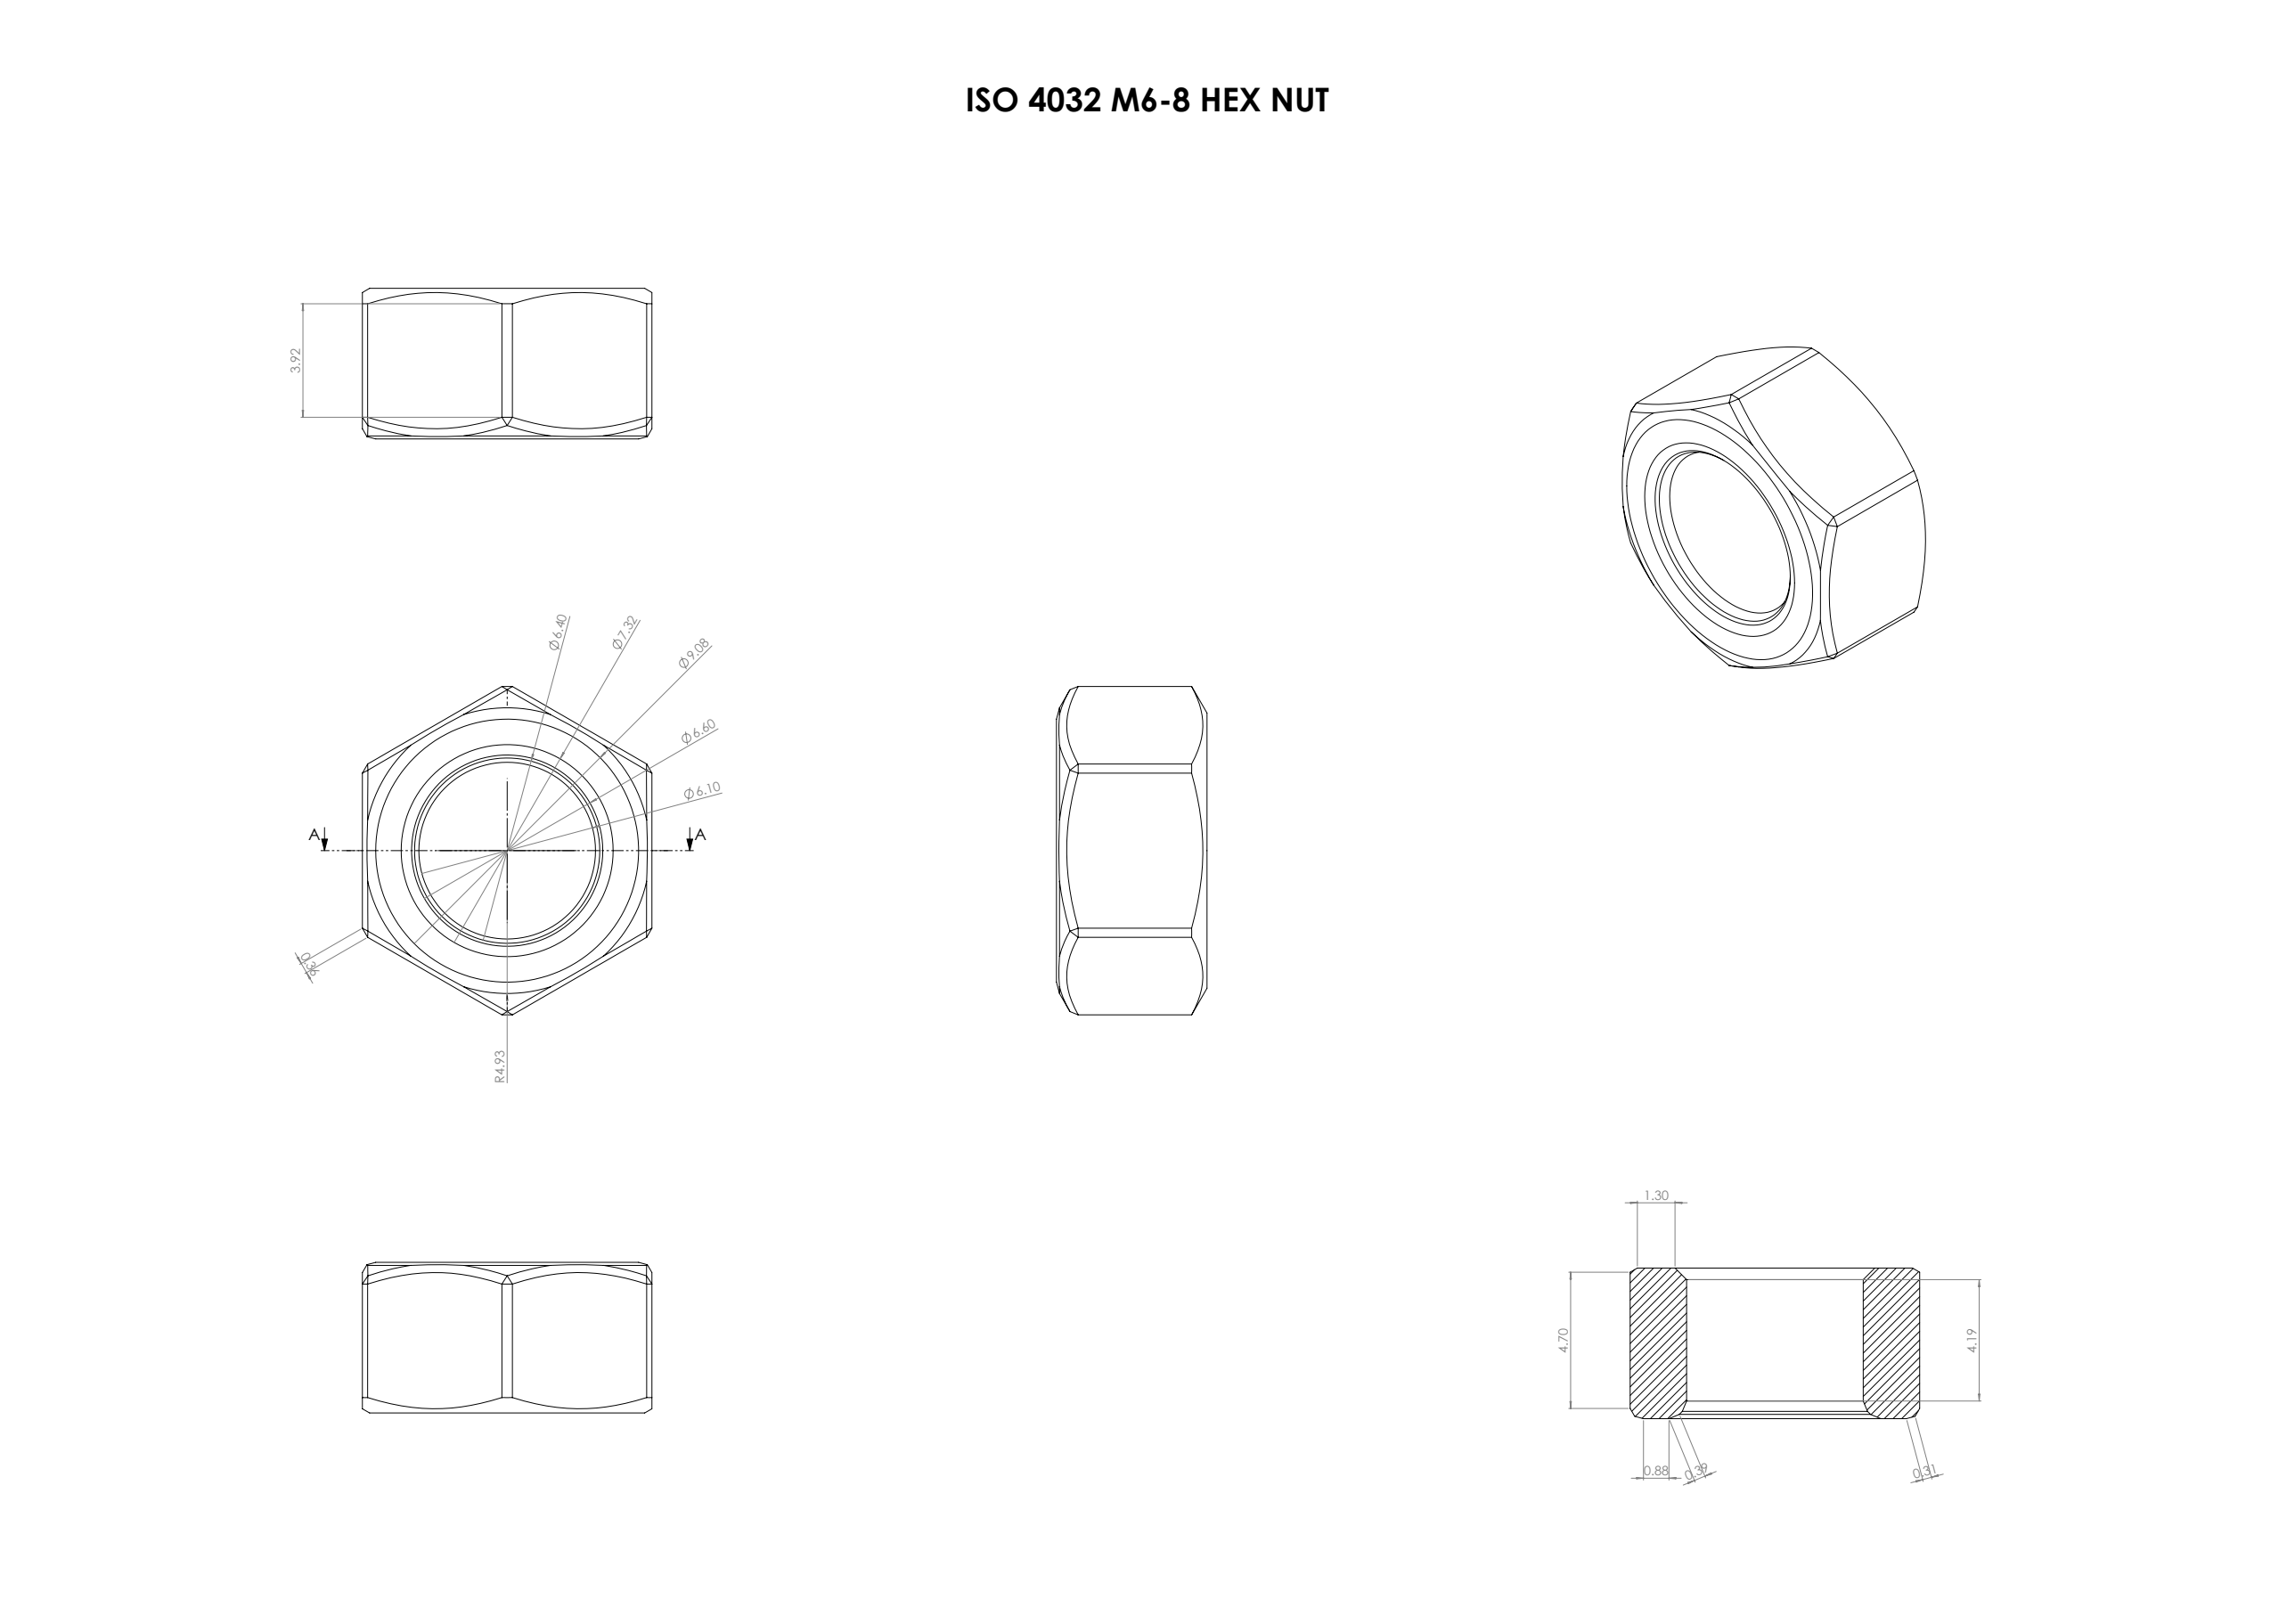
ISO-10303-21;
HEADER;
/* Generated by software containing ST-Developer
 * from STEP Tools, Inc. (www.steptools.com) 
 */

FILE_DESCRIPTION(
/* description */ (''),
/* implementation_level */ '2;1');

FILE_NAME(
/* name */ 
'11_ISO_4032_M6-8_Hex_Nut.step',
/* time_stamp */ '2026-10-22T00:21:42-07:00',
/* author */ (''),
/* organization */ (''),
/* preprocessor_version */ 'ST-DEVELOPER v20.2',
/* originating_system */ 'Autodesk Translation Framework v15.15.0.0',
/* authorisation */ '');

FILE_SCHEMA (('AUTOMOTIVE_DESIGN { 1 0 10303 214 3 1 1 }'));
ENDSEC;

DATA;
#10=MECHANICAL_DESIGN_GEOMETRIC_PRESENTATION_REPRESENTATION('',(#215),#31638);
#159=(
BOUNDED_CURVE()
B_SPLINE_CURVE(2,(#31154,#31155,#31156),.UNSPECIFIED.,.F.,.F.)
B_SPLINE_CURVE_WITH_KNOTS((3,3),(0.0913980941282311,0.128154684519473),
 .UNSPECIFIED.)
CURVE()
GEOMETRIC_REPRESENTATION_ITEM()
RATIONAL_B_SPLINE_CURVE((1.009002117709,1.00952129238835,1.009002117709))
REPRESENTATION_ITEM('')
);
#160=(
BOUNDED_CURVE()
B_SPLINE_CURVE(2,(#31282,#31283,#31284),.UNSPECIFIED.,.F.,.F.)
B_SPLINE_CURVE_WITH_KNOTS((3,3),(0.0913980941282308,0.128154684519473),
 .UNSPECIFIED.)
CURVE()
GEOMETRIC_REPRESENTATION_ITEM()
RATIONAL_B_SPLINE_CURVE((1.009002117709,1.00952129238836,1.009002117709))
REPRESENTATION_ITEM('')
);
#161=(
BOUNDED_CURVE()
B_SPLINE_CURVE(2,(#31290,#31291,#31292),.UNSPECIFIED.,.F.,.F.)
B_SPLINE_CURVE_WITH_KNOTS((3,3),(0.0913980941282322,0.128154684519474),
 .UNSPECIFIED.)
CURVE()
GEOMETRIC_REPRESENTATION_ITEM()
RATIONAL_B_SPLINE_CURVE((1.009002117709,1.00952129238836,1.009002117709))
REPRESENTATION_ITEM('')
);
#162=(
BOUNDED_CURVE()
B_SPLINE_CURVE(2,(#31423,#31424,#31425),.UNSPECIFIED.,.F.,.F.)
B_SPLINE_CURVE_WITH_KNOTS((3,3),(0.0913980941282321,0.128154684519474),
 .UNSPECIFIED.)
CURVE()
GEOMETRIC_REPRESENTATION_ITEM()
RATIONAL_B_SPLINE_CURVE((1.009002117709,1.00952129238835,1.009002117709))
REPRESENTATION_ITEM('')
);
#163=(
BOUNDED_CURVE()
B_SPLINE_CURVE(2,(#31431,#31432,#31433),.UNSPECIFIED.,.F.,.F.)
B_SPLINE_CURVE_WITH_KNOTS((3,3),(0.0913980941282314,0.128154684519474),
 .UNSPECIFIED.)
CURVE()
GEOMETRIC_REPRESENTATION_ITEM()
RATIONAL_B_SPLINE_CURVE((1.00900211770901,1.00952129238836,1.00900211770901))
REPRESENTATION_ITEM('')
);
#164=(
BOUNDED_CURVE()
B_SPLINE_CURVE(2,(#31499,#31500,#31501),.UNSPECIFIED.,.F.,.F.)
B_SPLINE_CURVE_WITH_KNOTS((3,3),(0.0913980941282296,0.128154684519472),
 .UNSPECIFIED.)
CURVE()
GEOMETRIC_REPRESENTATION_ITEM()
RATIONAL_B_SPLINE_CURVE((1.00900211770901,1.00952129238837,1.00900211770901))
REPRESENTATION_ITEM('')
);
#165=(
BOUNDED_CURVE()
B_SPLINE_CURVE(2,(#31505,#31506,#31507),.UNSPECIFIED.,.F.,.F.)
B_SPLINE_CURVE_WITH_KNOTS((3,3),(0.0979198359865813,0.674024179098759),
 .UNSPECIFIED.)
CURVE()
GEOMETRIC_REPRESENTATION_ITEM()
RATIONAL_B_SPLINE_CURVE((1.0564201716687,1.19828036671056,1.0564201716687))
REPRESENTATION_ITEM('')
);
#166=(
BOUNDED_CURVE()
B_SPLINE_CURVE(2,(#31509,#31510,#31511),.UNSPECIFIED.,.F.,.F.)
B_SPLINE_CURVE_WITH_KNOTS((3,3),(0.0979198359865817,0.674024179098759),
 .UNSPECIFIED.)
CURVE()
GEOMETRIC_REPRESENTATION_ITEM()
RATIONAL_B_SPLINE_CURVE((1.0564201716687,1.19828036671056,1.0564201716687))
REPRESENTATION_ITEM('')
);
#167=(
BOUNDED_CURVE()
B_SPLINE_CURVE(2,(#31513,#31514,#31515),.UNSPECIFIED.,.F.,.F.)
B_SPLINE_CURVE_WITH_KNOTS((3,3),(0.0979198359865813,0.674024179098759),
 .UNSPECIFIED.)
CURVE()
GEOMETRIC_REPRESENTATION_ITEM()
RATIONAL_B_SPLINE_CURVE((1.0564201716687,1.19828036671056,1.0564201716687))
REPRESENTATION_ITEM('')
);
#168=(
BOUNDED_CURVE()
B_SPLINE_CURVE(2,(#31521,#31522,#31523),.UNSPECIFIED.,.F.,.F.)
B_SPLINE_CURVE_WITH_KNOTS((3,3),(0.0979198359865812,0.385972007542669),
 .UNSPECIFIED.)
CURVE()
GEOMETRIC_REPRESENTATION_ITEM()
RATIONAL_B_SPLINE_CURVE((1.0564201716687,1.12735026918963,1.12735026918963))
REPRESENTATION_ITEM('')
);
#169=(
BOUNDED_CURVE()
B_SPLINE_CURVE(2,(#31524,#31525,#31526),.UNSPECIFIED.,.F.,.F.)
B_SPLINE_CURVE_WITH_KNOTS((3,3),(0.0979198359865812,0.674024179098759),
 .UNSPECIFIED.)
CURVE()
GEOMETRIC_REPRESENTATION_ITEM()
RATIONAL_B_SPLINE_CURVE((1.0564201716687,1.19828036671056,1.0564201716687))
REPRESENTATION_ITEM('')
);
#170=(
BOUNDED_CURVE()
B_SPLINE_CURVE(2,(#31527,#31528,#31529),.UNSPECIFIED.,.F.,.F.)
B_SPLINE_CURVE_WITH_KNOTS((3,3),(0.0979198359865813,0.674024179098759),
 .UNSPECIFIED.)
CURVE()
GEOMETRIC_REPRESENTATION_ITEM()
RATIONAL_B_SPLINE_CURVE((1.0564201716687,1.19828036671056,1.0564201716687))
REPRESENTATION_ITEM('')
);
#171=(
BOUNDED_CURVE()
B_SPLINE_CURVE(2,(#31530,#31531,#31532),.UNSPECIFIED.,.F.,.F.)
B_SPLINE_CURVE_WITH_KNOTS((3,3),(0.385972007542669,0.674024179098759),
 .UNSPECIFIED.)
CURVE()
GEOMETRIC_REPRESENTATION_ITEM()
RATIONAL_B_SPLINE_CURVE((1.12735026918963,1.12735026918963,1.0564201716687))
REPRESENTATION_ITEM('')
);
#193=SHAPE_REPRESENTATION_RELATIONSHIP('SRR','None',#31715,#204);
#204=ADVANCED_BREP_SHAPE_REPRESENTATION('',(#226),#31637);
#215=STYLED_ITEM('',(#31837),#226);
#226=MANIFOLD_SOLID_BREP('Hex nut',#12490);
#361=CYLINDRICAL_SURFACE('',#13575,0.305);
#445=CONICAL_SURFACE('',#13551,0.551175134594813,1.0471975511966);
#446=CONICAL_SURFACE('',#13553,0.551175134594813,1.0471975511966);
#447=CONICAL_SURFACE('',#13555,0.551175134594813,1.0471975511966);
#448=CONICAL_SURFACE('',#13557,0.551175134594813,1.0471975511966);
#449=CONICAL_SURFACE('',#13559,0.551175134594813,1.0471975511966);
#450=CONICAL_SURFACE('',#13561,0.551175134594813,1.0471975511966);
#451=CONICAL_SURFACE('',#13563,0.551175134594813,1.0471975511966);
#452=CONICAL_SURFACE('',#13565,0.473593266739736,1.30899693899575);
#453=CONICAL_SURFACE('',#13569,0.348075378797541,1.17809724509617);
#454=CONICAL_SURFACE('',#13571,0.325,0.785398163397448);
#455=CONICAL_SURFACE('',#13573,0.312424621202459,0.392699081698723);
#456=CONICAL_SURFACE('',#13577,0.325,0.785398163397448);
#1149=B_SPLINE_CURVE_WITH_KNOTS('',3,(#30994,#30995,#30996,#30997,#30998,
#30999),.UNSPECIFIED.,.F.,.F.,(4,2,4),(-0.0356445426705879,-0.017820065955887,
0.),.UNSPECIFIED.);
#1150=B_SPLINE_CURVE_WITH_KNOTS('',3,(#31000,#31001,#31002,#31003,#31004,
#31005),.UNSPECIFIED.,.F.,.F.,(4,2,4),(-0.0356445406593133,-0.0178242377363697,
0.),.UNSPECIFIED.);
#1151=B_SPLINE_CURVE_WITH_KNOTS('',3,(#31009,#31010,#31011,#31012,#31013,
#31014),.UNSPECIFIED.,.F.,.F.,(4,2,4),(-0.0356445426646998,-0.0178200659542505,
0.),.UNSPECIFIED.);
#1152=B_SPLINE_CURVE_WITH_KNOTS('',3,(#31016,#31017,#31018,#31019,#31020,
#31021),.UNSPECIFIED.,.F.,.F.,(4,2,4),(-0.0356445406608173,-0.0178242377372387,
0.),.UNSPECIFIED.);
#1153=B_SPLINE_CURVE_WITH_KNOTS('',3,(#31028,#31029,#31030,#31031,#31032,
#31033),.UNSPECIFIED.,.F.,.F.,(4,2,4),(-0.035644542668606,-0.0178200659552084,
0.),.UNSPECIFIED.);
#1154=B_SPLINE_CURVE_WITH_KNOTS('',3,(#31034,#31035,#31036,#31037,#31038,
#31039),.UNSPECIFIED.,.F.,.F.,(4,2,4),(-0.0356445406611976,-0.0178242377369016,
0.),.UNSPECIFIED.);
#1155=B_SPLINE_CURVE_WITH_KNOTS('',3,(#31043,#31044,#31045,#31046,#31047,
#31048),.UNSPECIFIED.,.F.,.F.,(4,2,4),(-0.0356445426695261,-0.0178200659558121,
0.),.UNSPECIFIED.);
#1156=B_SPLINE_CURVE_WITH_KNOTS('',3,(#31050,#31051,#31052,#31053,#31054,
#31055),.UNSPECIFIED.,.F.,.F.,(4,2,4),(-0.0356445406606661,-0.0178242377367645,
0.),.UNSPECIFIED.);
#1157=B_SPLINE_CURVE_WITH_KNOTS('',3,(#31062,#31063,#31064,#31065,#31066,
#31067),.UNSPECIFIED.,.F.,.F.,(4,2,4),(-0.0356445426677898,-0.0178200659551202,
0.),.UNSPECIFIED.);
#1158=B_SPLINE_CURVE_WITH_KNOTS('',3,(#31068,#31069,#31070,#31071,#31072,
#31073),.UNSPECIFIED.,.F.,.F.,(4,2,4),(-0.0356445406615696,-0.0178242377363734,
0.),.UNSPECIFIED.);
#1159=B_SPLINE_CURVE_WITH_KNOTS('',3,(#31077,#31078,#31079,#31080,#31081,
#31082),.UNSPECIFIED.,.F.,.F.,(4,2,4),(-0.0356445426680788,-0.017820065955108,
0.),.UNSPECIFIED.);
#1160=B_SPLINE_CURVE_WITH_KNOTS('',3,(#31084,#31085,#31086,#31087,#31088,
#31089),.UNSPECIFIED.,.F.,.F.,(4,2,4),(-0.0356445406623922,-0.0178242377374904,
0.),.UNSPECIFIED.);
#1161=B_SPLINE_CURVE_WITH_KNOTS('',3,(#31113,#31114,#31115,#31116,#31117,
#31118,#31119,#31120,#31121,#31122,#31123,#31124,#31125,#31126,#31127,#31128,
#31129,#31130,#31131,#31132,#31133,#31134,#31135,#31136,#31137),
 .UNSPECIFIED.,.F.,.F.,(4,3,3,3,3,3,3,3,4),(1.38777878078145E-17,0.0499520104369165,
0.0579096339663456,0.0689507685252385,0.0901012807338169,0.116325803406286,
0.146260951142593,0.196900647008064,0.212043967873001),.UNSPECIFIED.);
#1162=B_SPLINE_CURVE_WITH_KNOTS('',3,(#31138,#31139,#31140,#31141),
 .UNSPECIFIED.,.F.,.F.,(4,4),(0.50492078692473,0.681229914591334),
 .UNSPECIFIED.);
#1163=B_SPLINE_CURVE_WITH_KNOTS('',3,(#31142,#31143,#31144,#31145,#31146),
 .UNSPECIFIED.,.F.,.F.,(4,1,4),(-0.679321786705464,-0.343792306535718,-0.0926222283799249),
 .UNSPECIFIED.);
#1164=B_SPLINE_CURVE_WITH_KNOTS('',3,(#31147,#31148,#31149,#31150),
 .UNSPECIFIED.,.F.,.F.,(4,4),(0.0907141004940068,0.26702322816061),
 .UNSPECIFIED.);
#1165=B_SPLINE_CURVE_WITH_KNOTS('',3,(#31181,#31182,#31183,#31184,#31185,
#31186,#31187,#31188,#31189,#31190,#31191,#31192,#31193,#31194,#31195,#31196,
#31197,#31198,#31199,#31200,#31201,#31202,#31203,#31204,#31205),
 .UNSPECIFIED.,.F.,.F.,(4,3,3,3,3,3,3,3,4),(0.,0.0499552658273372,0.0579096339663306,
0.0689507685252128,0.0901012807337863,0.116325803406243,0.146260951142533,
0.196900647007959,0.212043967872853),.UNSPECIFIED.);
#1166=B_SPLINE_CURVE_WITH_KNOTS('',3,(#31206,#31207,#31208,#31209),
 .UNSPECIFIED.,.F.,.F.,(4,4),(0.504920786924729,0.681229914591334),
 .UNSPECIFIED.);
#1167=B_SPLINE_CURVE_WITH_KNOTS('',3,(#31210,#31211,#31212,#31213,#31214),
 .UNSPECIFIED.,.F.,.F.,(4,1,4),(-0.679321786705464,-0.343792306535718,-0.092622228379925),
 .UNSPECIFIED.);
#1168=B_SPLINE_CURVE_WITH_KNOTS('',3,(#31215,#31216,#31217,#31218),
 .UNSPECIFIED.,.F.,.F.,(4,4),(0.0907141004940068,0.26702322816061),
 .UNSPECIFIED.);
#1169=B_SPLINE_CURVE_WITH_KNOTS('',3,(#31241,#31242,#31243,#31244,#31245,
#31246,#31247,#31248,#31249,#31250,#31251,#31252,#31253,#31254,#31255,#31256,
#31257,#31258,#31259,#31260,#31261,#31262,#31263,#31264,#31265),
 .UNSPECIFIED.,.F.,.F.,(4,3,3,3,3,3,3,3,4),(0.,0.0499520104360042,0.0579096339663052,
0.0689507685251914,0.0901012807337567,0.116325803406213,0.14626095114252,
0.196900647008034,0.212043967872961),.UNSPECIFIED.);
#1170=B_SPLINE_CURVE_WITH_KNOTS('',3,(#31266,#31267,#31268,#31269),
 .UNSPECIFIED.,.F.,.F.,(4,4),(0.50492078692473,0.681229914591334),
 .UNSPECIFIED.);
#1171=B_SPLINE_CURVE_WITH_KNOTS('',3,(#31270,#31271,#31272,#31273,#31274),
 .UNSPECIFIED.,.F.,.F.,(4,1,4),(-0.679321786705465,-0.343792306535719,-0.092622228379925),
 .UNSPECIFIED.);
#1172=B_SPLINE_CURVE_WITH_KNOTS('',3,(#31275,#31276,#31277,#31278),
 .UNSPECIFIED.,.F.,.F.,(4,4),(0.0907141004940071,0.26702322816061),
 .UNSPECIFIED.);
#1173=B_SPLINE_CURVE_WITH_KNOTS('',3,(#31317,#31318,#31319,#31320,#31321,
#31322,#31323,#31324,#31325,#31326,#31327,#31328,#31329,#31330,#31331,#31332,
#31333,#31334,#31335,#31336,#31337,#31338,#31339,#31340,#31341),
 .UNSPECIFIED.,.F.,.F.,(4,3,3,3,3,3,3,3,4),(0.,0.0501067129681924,0.0579096339662997,
0.0901012807337445,0.116325803406229,0.14310556044029,0.146260951142586,
0.196900647008164,0.212043967873065),.UNSPECIFIED.);
#1174=B_SPLINE_CURVE_WITH_KNOTS('',3,(#31342,#31343,#31344,#31345),
 .UNSPECIFIED.,.F.,.F.,(4,4),(0.50492078692473,0.681229914591334),
 .UNSPECIFIED.);
#1175=B_SPLINE_CURVE_WITH_KNOTS('',3,(#31346,#31347,#31348,#31349,#31350),
 .UNSPECIFIED.,.F.,.F.,(4,1,4),(-0.679321786705464,-0.428151708549622,-0.0926222283799251),
 .UNSPECIFIED.);
#1176=B_SPLINE_CURVE_WITH_KNOTS('',3,(#31351,#31352,#31353,#31354),
 .UNSPECIFIED.,.F.,.F.,(4,4),(0.0907141004940069,0.267023228160609),
 .UNSPECIFIED.);
#1177=B_SPLINE_CURVE_WITH_KNOTS('',3,(#31377,#31378,#31379,#31380,#31381,
#31382,#31383,#31384,#31385,#31386,#31387,#31388,#31389),.UNSPECIFIED.,
 .F.,.F.,(4,3,3,3,4),(0.,0.050107747114841,0.0579096339663157,0.0901012807337753,
0.106028581745725),.UNSPECIFIED.);
#1178=B_SPLINE_CURVE_WITH_KNOTS('',3,(#31391,#31392,#31393,#31394,#31395,
#31396,#31397,#31398,#31399,#31400,#31401,#31402,#31403,#31404,#31405,#31406),
 .UNSPECIFIED.,.F.,.F.,(4,3,3,3,3,4),(0.106028581745725,0.11632580340628,
0.143105560440363,0.146260951142647,0.196900647008195,0.212043967873119),
 .UNSPECIFIED.);
#1179=B_SPLINE_CURVE_WITH_KNOTS('',3,(#31407,#31408,#31409,#31410),
 .UNSPECIFIED.,.F.,.F.,(4,4),(0.50492078692473,0.681229914591334),
 .UNSPECIFIED.);
#1180=B_SPLINE_CURVE_WITH_KNOTS('',3,(#31411,#31412,#31413,#31414,#31415),
 .UNSPECIFIED.,.F.,.F.,(4,1,4),(-0.679321786705464,-0.428151708549622,-0.0926222283799252),
 .UNSPECIFIED.);
#1181=B_SPLINE_CURVE_WITH_KNOTS('',3,(#31416,#31417,#31418,#31419),
 .UNSPECIFIED.,.F.,.F.,(4,4),(0.090714100494007,0.26702322816061),
 .UNSPECIFIED.);
#1182=B_SPLINE_CURVE_WITH_KNOTS('',3,(#31458,#31459,#31460,#31461,#31462,
#31463,#31464,#31465,#31466,#31467,#31468,#31469,#31470,#31471,#31472,#31473,
#31474,#31475,#31476,#31477,#31478,#31479,#31480,#31481,#31482),
 .UNSPECIFIED.,.F.,.F.,(4,3,3,3,3,3,3,3,4),(0.,0.0499520104361464,0.0579096339662874,
0.0689507685251644,0.0901012807337523,0.116325803406236,0.146260951142573,
0.196900647008118,0.21204396787299),.UNSPECIFIED.);
#1183=B_SPLINE_CURVE_WITH_KNOTS('',3,(#31483,#31484,#31485,#31486),
 .UNSPECIFIED.,.F.,.F.,(4,4),(0.504920786924729,0.681229914591334),
 .UNSPECIFIED.);
#1184=B_SPLINE_CURVE_WITH_KNOTS('',3,(#31487,#31488,#31489,#31490,#31491),
 .UNSPECIFIED.,.F.,.F.,(4,1,4),(-0.679321786705464,-0.343792306535719,-0.0926222283799251),
 .UNSPECIFIED.);
#1185=B_SPLINE_CURVE_WITH_KNOTS('',3,(#31492,#31493,#31494,#31495),
 .UNSPECIFIED.,.F.,.F.,(4,4),(0.0907141004940075,0.26702322816061),
 .UNSPECIFIED.);
#1334=B_SPLINE_SURFACE_WITH_KNOTS('',3,3,((#31091,#31092,#31093,#31094,
#31095),(#31096,#31097,#31098,#31099,#31100),(#31101,#31102,#31103,#31104,
#31105),(#31106,#31107,#31108,#31109,#31110)),.UNSPECIFIED.,.F.,.F.,.F.,
(4,4),(4,1,4),(0.,1.),(0.0907141004940068,0.343792306535718,0.681229914591334),
 .UNSPECIFIED.);
#1335=B_SPLINE_SURFACE_WITH_KNOTS('',3,3,((#31159,#31160,#31161,#31162,
#31163),(#31164,#31165,#31166,#31167,#31168),(#31169,#31170,#31171,#31172,
#31173),(#31174,#31175,#31176,#31177,#31178)),.UNSPECIFIED.,.F.,.F.,.F.,
(4,4),(4,1,4),(0.,1.),(0.0907141004940068,0.343792306535718,0.681229914591334),
 .UNSPECIFIED.);
#1336=B_SPLINE_SURFACE_WITH_KNOTS('',3,3,((#31219,#31220,#31221,#31222,
#31223),(#31224,#31225,#31226,#31227,#31228),(#31229,#31230,#31231,#31232,
#31233),(#31234,#31235,#31236,#31237,#31238)),.UNSPECIFIED.,.F.,.F.,.F.,
(4,4),(4,1,4),(0.,1.),(0.0907141004940071,0.343792306535719,0.681229914591334),
 .UNSPECIFIED.);
#1337=B_SPLINE_SURFACE_WITH_KNOTS('',3,3,((#31295,#31296,#31297,#31298,
#31299),(#31300,#31301,#31302,#31303,#31304),(#31305,#31306,#31307,#31308,
#31309),(#31310,#31311,#31312,#31313,#31314)),.UNSPECIFIED.,.F.,.F.,.F.,
(4,4),(4,1,4),(0.,1.),(0.0907141004940069,0.428151708549622,0.681229914591334),
 .UNSPECIFIED.);
#1338=B_SPLINE_SURFACE_WITH_KNOTS('',3,3,((#31355,#31356,#31357,#31358,
#31359),(#31360,#31361,#31362,#31363,#31364),(#31365,#31366,#31367,#31368,
#31369),(#31370,#31371,#31372,#31373,#31374)),.UNSPECIFIED.,.F.,.F.,.F.,
(4,4),(4,1,4),(0.,1.),(0.090714100494007,0.428151708549622,0.681229914591334),
 .UNSPECIFIED.);
#1339=B_SPLINE_SURFACE_WITH_KNOTS('',3,3,((#31436,#31437,#31438,#31439,
#31440),(#31441,#31442,#31443,#31444,#31445),(#31446,#31447,#31448,#31449,
#31450),(#31451,#31452,#31453,#31454,#31455)),.UNSPECIFIED.,.F.,.F.,.F.,
(4,4),(4,1,4),(0.,1.),(0.0907141004940075,0.343792306535719,0.681229914591334),
 .UNSPECIFIED.);
#1403=FACE_BOUND('',#3261,.T.);
#1404=FACE_BOUND('',#3268,.T.);
#1805=CIRCLE('',#13552,0.475);
#1806=CIRCLE('',#13554,0.493186533479473);
#1807=CIRCLE('',#13556,0.493186533479473);
#1808=CIRCLE('',#13558,0.493186533479473);
#1809=CIRCLE('',#13560,0.493186533479473);
#1810=CIRCLE('',#13562,0.493186533479473);
#1811=CIRCLE('',#13564,0.493186533479473);
#1812=CIRCLE('',#13566,0.454);
#1813=CIRCLE('',#13568,0.366);
#1814=CIRCLE('',#13570,0.330150757595083);
#1815=CIRCLE('',#13572,0.319849242404917);
#1816=CIRCLE('',#13574,0.305);
#1817=CIRCLE('',#13576,0.305);
#1818=CIRCLE('',#13578,0.345);
#2474=FACE_OUTER_BOUND('',#3231,.T.);
#2475=FACE_OUTER_BOUND('',#3232,.T.);
#2476=FACE_OUTER_BOUND('',#3233,.T.);
#2477=FACE_OUTER_BOUND('',#3234,.T.);
#2478=FACE_OUTER_BOUND('',#3235,.T.);
#2479=FACE_OUTER_BOUND('',#3236,.T.);
#2480=FACE_OUTER_BOUND('',#3237,.T.);
#2481=FACE_OUTER_BOUND('',#3238,.T.);
#2482=FACE_OUTER_BOUND('',#3239,.T.);
#2483=FACE_OUTER_BOUND('',#3240,.T.);
#2484=FACE_OUTER_BOUND('',#3241,.T.);
#2485=FACE_OUTER_BOUND('',#3242,.T.);
#2486=FACE_OUTER_BOUND('',#3243,.T.);
#2487=FACE_OUTER_BOUND('',#3244,.T.);
#2488=FACE_OUTER_BOUND('',#3245,.T.);
#2489=FACE_OUTER_BOUND('',#3246,.T.);
#2490=FACE_OUTER_BOUND('',#3247,.T.);
#2491=FACE_OUTER_BOUND('',#3248,.T.);
#2492=FACE_OUTER_BOUND('',#3249,.T.);
#2493=FACE_OUTER_BOUND('',#3250,.T.);
#2494=FACE_OUTER_BOUND('',#3251,.T.);
#2495=FACE_OUTER_BOUND('',#3252,.T.);
#2496=FACE_OUTER_BOUND('',#3253,.T.);
#2497=FACE_OUTER_BOUND('',#3254,.T.);
#2498=FACE_OUTER_BOUND('',#3255,.T.);
#2499=FACE_OUTER_BOUND('',#3256,.T.);
#2500=FACE_OUTER_BOUND('',#3257,.T.);
#2501=FACE_OUTER_BOUND('',#3258,.T.);
#2502=FACE_OUTER_BOUND('',#3259,.T.);
#2503=FACE_OUTER_BOUND('',#3260,.T.);
#2504=FACE_OUTER_BOUND('',#3262,.T.);
#2505=FACE_OUTER_BOUND('',#3263,.T.);
#2506=FACE_OUTER_BOUND('',#3264,.T.);
#2507=FACE_OUTER_BOUND('',#3265,.T.);
#2508=FACE_OUTER_BOUND('',#3266,.T.);
#2509=FACE_OUTER_BOUND('',#3267,.T.);
#2510=FACE_OUTER_BOUND('',#3269,.T.);
#2511=FACE_OUTER_BOUND('',#3270,.T.);
#2512=FACE_OUTER_BOUND('',#3271,.T.);
#3231=EDGE_LOOP('',(#11305,#11306,#11307));
#3232=EDGE_LOOP('',(#11308,#11309,#11310));
#3233=EDGE_LOOP('',(#11311,#11312,#11313));
#3234=EDGE_LOOP('',(#11314,#11315,#11316));
#3235=EDGE_LOOP('',(#11317,#11318,#11319));
#3236=EDGE_LOOP('',(#11320,#11321,#11322));
#3237=EDGE_LOOP('',(#11323,#11324,#11325,#11326,#11327,#11328));
#3238=EDGE_LOOP('',(#11329,#11330,#11331,#11332));
#3239=EDGE_LOOP('',(#11333,#11334,#11335,#11336,#11337,#11338));
#3240=EDGE_LOOP('',(#11339,#11340,#11341,#11342,#11343,#11344));
#3241=EDGE_LOOP('',(#11345,#11346,#11347,#11348));
#3242=EDGE_LOOP('',(#11349,#11350,#11351,#11352));
#3243=EDGE_LOOP('',(#11353,#11354,#11355,#11356,#11357,#11358));
#3244=EDGE_LOOP('',(#11359,#11360,#11361,#11362,#11363,#11364,#11365));
#3245=EDGE_LOOP('',(#11366,#11367,#11368,#11369));
#3246=EDGE_LOOP('',(#11370,#11371,#11372,#11373));
#3247=EDGE_LOOP('',(#11374,#11375,#11376,#11377,#11378,#11379));
#3248=EDGE_LOOP('',(#11380,#11381,#11382,#11383));
#3249=EDGE_LOOP('',(#11384,#11385,#11386,#11387));
#3250=EDGE_LOOP('',(#11388,#11389,#11390,#11391));
#3251=EDGE_LOOP('',(#11392,#11393,#11394,#11395));
#3252=EDGE_LOOP('',(#11396,#11397,#11398,#11399,#11400,#11401,#11402,#11403,
#11404,#11405,#11406,#11407,#11408,#11409,#11410,#11411));
#3253=EDGE_LOOP('',(#11412,#11413,#11414));
#3254=EDGE_LOOP('',(#11415,#11416,#11417));
#3255=EDGE_LOOP('',(#11418,#11419,#11420));
#3256=EDGE_LOOP('',(#11421,#11422,#11423));
#3257=EDGE_LOOP('',(#11424,#11425,#11426));
#3258=EDGE_LOOP('',(#11427,#11428,#11429));
#3259=EDGE_LOOP('',(#11430,#11431,#11432,#11433,#11434,#11435,#11436,#11437,
#11438,#11439,#11440,#11441,#11442,#11443,#11444,#11445));
#3260=EDGE_LOOP('',(#11446));
#3261=EDGE_LOOP('',(#11447));
#3262=EDGE_LOOP('',(#11448,#11449,#11450,#11451));
#3263=EDGE_LOOP('',(#11452,#11453,#11454,#11455));
#3264=EDGE_LOOP('',(#11456,#11457,#11458,#11459));
#3265=EDGE_LOOP('',(#11460,#11461,#11462,#11463));
#3266=EDGE_LOOP('',(#11464,#11465,#11466,#11467));
#3267=EDGE_LOOP('',(#11468));
#3268=EDGE_LOOP('',(#11469));
#3269=EDGE_LOOP('',(#11470,#11471,#11472,#11473));
#3270=EDGE_LOOP('',(#11474,#11475,#11476,#11477,#11478));
#3271=EDGE_LOOP('',(#11479,#11480,#11481,#11482));
#3952=LINE('',#30992,#4657);
#3953=LINE('',#31022,#4658);
#3954=LINE('',#31026,#4659);
#3955=LINE('',#31056,#4660);
#3956=LINE('',#31060,#4661);
#3957=LINE('',#31090,#4662);
#3958=LINE('',#31157,#4663);
#3959=LINE('',#31158,#4664);
#3960=LINE('',#31285,#4665);
#3961=LINE('',#31286,#4666);
#3962=LINE('',#31293,#4667);
#3963=LINE('',#31294,#4668);
#3964=LINE('',#31426,#4669);
#3965=LINE('',#31427,#4670);
#3966=LINE('',#31434,#4671);
#3967=LINE('',#31435,#4672);
#3968=LINE('',#31502,#4673);
#3969=LINE('',#31503,#4674);
#3970=LINE('',#31520,#4675);
#3971=LINE('',#31548,#4676);
#3972=LINE('',#31555,#4677);
#3973=LINE('',#31558,#4678);
#3974=LINE('',#31562,#4679);
#3975=LINE('',#31566,#4680);
#3976=LINE('',#31570,#4681);
#4657=VECTOR('',#16148,1.);
#4658=VECTOR('',#16151,1.);
#4659=VECTOR('',#16154,1.);
#4660=VECTOR('',#16157,1.);
#4661=VECTOR('',#16160,1.);
#4662=VECTOR('',#16163,1.);
#4663=VECTOR('',#16166,1.);
#4664=VECTOR('',#16167,1.);
#4665=VECTOR('',#16170,1.);
#4666=VECTOR('',#16171,1.);
#4667=VECTOR('',#16174,1.);
#4668=VECTOR('',#16175,1.);
#4669=VECTOR('',#16178,1.);
#4670=VECTOR('',#16179,1.);
#4671=VECTOR('',#16182,1.);
#4672=VECTOR('',#16183,1.);
#4673=VECTOR('',#16186,1.);
#4674=VECTOR('',#16187,1.);
#4675=VECTOR('',#16198,0.551175134594813);
#4676=VECTOR('',#16227,0.473593266739737);
#4677=VECTOR('',#16236,0.348075378797541);
#4678=VECTOR('',#16239,0.325);
#4679=VECTOR('',#16244,0.312424621202459);
#4680=VECTOR('',#16249,0.305);
#4681=VECTOR('',#16254,0.325);
#5836=VERTEX_POINT('',#30990);
#5837=VERTEX_POINT('',#30991);
#5838=VERTEX_POINT('',#30993);
#5839=VERTEX_POINT('',#31007);
#5840=VERTEX_POINT('',#31008);
#5841=VERTEX_POINT('',#31015);
#5842=VERTEX_POINT('',#31024);
#5843=VERTEX_POINT('',#31025);
#5844=VERTEX_POINT('',#31027);
#5845=VERTEX_POINT('',#31041);
#5846=VERTEX_POINT('',#31042);
#5847=VERTEX_POINT('',#31049);
#5848=VERTEX_POINT('',#31058);
#5849=VERTEX_POINT('',#31059);
#5850=VERTEX_POINT('',#31061);
#5851=VERTEX_POINT('',#31075);
#5852=VERTEX_POINT('',#31076);
#5853=VERTEX_POINT('',#31083);
#5854=VERTEX_POINT('',#31111);
#5855=VERTEX_POINT('',#31112);
#5856=VERTEX_POINT('',#31152);
#5857=VERTEX_POINT('',#31153);
#5858=VERTEX_POINT('',#31179);
#5859=VERTEX_POINT('',#31180);
#5860=VERTEX_POINT('',#31239);
#5861=VERTEX_POINT('',#31240);
#5862=VERTEX_POINT('',#31280);
#5863=VERTEX_POINT('',#31281);
#5864=VERTEX_POINT('',#31288);
#5865=VERTEX_POINT('',#31289);
#5866=VERTEX_POINT('',#31315);
#5867=VERTEX_POINT('',#31316);
#5868=VERTEX_POINT('',#31375);
#5869=VERTEX_POINT('',#31376);
#5870=VERTEX_POINT('',#31390);
#5871=VERTEX_POINT('',#31421);
#5872=VERTEX_POINT('',#31422);
#5873=VERTEX_POINT('',#31429);
#5874=VERTEX_POINT('',#31430);
#5875=VERTEX_POINT('',#31456);
#5876=VERTEX_POINT('',#31457);
#5877=VERTEX_POINT('',#31497);
#5878=VERTEX_POINT('',#31498);
#5879=VERTEX_POINT('',#31517);
#5880=VERTEX_POINT('',#31519);
#5881=VERTEX_POINT('',#31546);
#5882=VERTEX_POINT('',#31550);
#5883=VERTEX_POINT('',#31553);
#5884=VERTEX_POINT('',#31557);
#5885=VERTEX_POINT('',#31561);
#5886=VERTEX_POINT('',#31565);
#5887=VERTEX_POINT('',#31569);
#7664=EDGE_CURVE('',#5836,#5837,#3952,.T.);
#7665=EDGE_CURVE('',#5838,#5836,#1149,.F.);
#7666=EDGE_CURVE('',#5837,#5838,#1150,.F.);
#7667=EDGE_CURVE('',#5839,#5840,#1151,.F.);
#7668=EDGE_CURVE('',#5841,#5839,#1152,.F.);
#7669=EDGE_CURVE('',#5840,#5841,#3953,.T.);
#7670=EDGE_CURVE('',#5842,#5843,#3954,.T.);
#7671=EDGE_CURVE('',#5844,#5842,#1153,.F.);
#7672=EDGE_CURVE('',#5843,#5844,#1154,.F.);
#7673=EDGE_CURVE('',#5845,#5846,#1155,.F.);
#7674=EDGE_CURVE('',#5847,#5845,#1156,.F.);
#7675=EDGE_CURVE('',#5846,#5847,#3955,.T.);
#7676=EDGE_CURVE('',#5848,#5849,#3956,.T.);
#7677=EDGE_CURVE('',#5850,#5848,#1157,.F.);
#7678=EDGE_CURVE('',#5849,#5850,#1158,.F.);
#7679=EDGE_CURVE('',#5851,#5852,#1159,.F.);
#7680=EDGE_CURVE('',#5853,#5851,#1160,.F.);
#7681=EDGE_CURVE('',#5852,#5853,#3957,.T.);
#7682=EDGE_CURVE('',#5854,#5855,#1161,.T.);
#7683=EDGE_CURVE('',#5855,#5850,#1162,.T.);
#7684=EDGE_CURVE('',#5848,#5853,#1163,.T.);
#7685=EDGE_CURVE('',#5851,#5854,#1164,.T.);
#7686=EDGE_CURVE('',#5856,#5857,#159,.T.);
#7687=EDGE_CURVE('',#5857,#5852,#3958,.T.);
#7688=EDGE_CURVE('',#5853,#5856,#3959,.T.);
#7689=EDGE_CURVE('',#5858,#5859,#1165,.T.);
#7690=EDGE_CURVE('',#5859,#5851,#1166,.T.);
#7691=EDGE_CURVE('',#5852,#5847,#1167,.T.);
#7692=EDGE_CURVE('',#5845,#5858,#1168,.T.);
#7693=EDGE_CURVE('',#5860,#5861,#1169,.T.);
#7694=EDGE_CURVE('',#5861,#5844,#1170,.T.);
#7695=EDGE_CURVE('',#5842,#5849,#1171,.T.);
#7696=EDGE_CURVE('',#5850,#5860,#1172,.T.);
#7697=EDGE_CURVE('',#5862,#5863,#160,.T.);
#7698=EDGE_CURVE('',#5863,#5848,#3960,.T.);
#7699=EDGE_CURVE('',#5849,#5862,#3961,.T.);
#7700=EDGE_CURVE('',#5864,#5865,#161,.T.);
#7701=EDGE_CURVE('',#5865,#5846,#3962,.T.);
#7702=EDGE_CURVE('',#5847,#5864,#3963,.T.);
#7703=EDGE_CURVE('',#5866,#5867,#1173,.T.);
#7704=EDGE_CURVE('',#5867,#5845,#1174,.T.);
#7705=EDGE_CURVE('',#5846,#5841,#1175,.T.);
#7706=EDGE_CURVE('',#5839,#5866,#1176,.T.);
#7707=EDGE_CURVE('',#5868,#5869,#1177,.T.);
#7708=EDGE_CURVE('',#5869,#5870,#1178,.T.);
#7709=EDGE_CURVE('',#5870,#5838,#1179,.T.);
#7710=EDGE_CURVE('',#5836,#5843,#1180,.T.);
#7711=EDGE_CURVE('',#5844,#5868,#1181,.T.);
#7712=EDGE_CURVE('',#5871,#5872,#162,.T.);
#7713=EDGE_CURVE('',#5872,#5842,#3964,.T.);
#7714=EDGE_CURVE('',#5843,#5871,#3965,.T.);
#7715=EDGE_CURVE('',#5873,#5874,#163,.T.);
#7716=EDGE_CURVE('',#5874,#5840,#3966,.T.);
#7717=EDGE_CURVE('',#5841,#5873,#3967,.T.);
#7718=EDGE_CURVE('',#5875,#5876,#1182,.T.);
#7719=EDGE_CURVE('',#5876,#5839,#1183,.T.);
#7720=EDGE_CURVE('',#5840,#5837,#1184,.T.);
#7721=EDGE_CURVE('',#5838,#5875,#1185,.T.);
#7722=EDGE_CURVE('',#5877,#5878,#164,.T.);
#7723=EDGE_CURVE('',#5878,#5836,#3968,.T.);
#7724=EDGE_CURVE('',#5837,#5877,#3969,.T.);
#7725=EDGE_CURVE('',#5872,#5862,#165,.T.);
#7726=EDGE_CURVE('',#5878,#5871,#166,.T.);
#7727=EDGE_CURVE('',#5874,#5877,#167,.T.);
#7728=EDGE_CURVE('',#5879,#5879,#1805,.T.);
#7729=EDGE_CURVE('',#5879,#5880,#3970,.T.);
#7730=EDGE_CURVE('',#5857,#5880,#168,.T.);
#7731=EDGE_CURVE('',#5863,#5856,#169,.T.);
#7732=EDGE_CURVE('',#5865,#5873,#170,.T.);
#7733=EDGE_CURVE('',#5880,#5864,#171,.T.);
#7734=EDGE_CURVE('',#5858,#5867,#1806,.T.);
#7735=EDGE_CURVE('',#5866,#5876,#1807,.T.);
#7736=EDGE_CURVE('',#5875,#5870,#1808,.T.);
#7737=EDGE_CURVE('',#5868,#5861,#1809,.T.);
#7738=EDGE_CURVE('',#5860,#5855,#1810,.T.);
#7739=EDGE_CURVE('',#5854,#5859,#1811,.T.);
#7740=EDGE_CURVE('',#5881,#5881,#1812,.T.);
#7741=EDGE_CURVE('',#5881,#5869,#3971,.T.);
#7742=EDGE_CURVE('',#5882,#5882,#1813,.T.);
#7743=EDGE_CURVE('',#5883,#5883,#1814,.T.);
#7744=EDGE_CURVE('',#5883,#5882,#3972,.T.);
#7745=EDGE_CURVE('',#5883,#5884,#3973,.T.);
#7746=EDGE_CURVE('',#5884,#5884,#1815,.T.);
#7747=EDGE_CURVE('',#5884,#5885,#3974,.T.);
#7748=EDGE_CURVE('',#5885,#5885,#1816,.T.);
#7749=EDGE_CURVE('',#5885,#5886,#3975,.T.);
#7750=EDGE_CURVE('',#5886,#5886,#1817,.T.);
#7751=EDGE_CURVE('',#5886,#5887,#3976,.T.);
#7752=EDGE_CURVE('',#5887,#5887,#1818,.T.);
#11305=ORIENTED_EDGE('',*,*,#7664,.F.);
#11306=ORIENTED_EDGE('',*,*,#7665,.F.);
#11307=ORIENTED_EDGE('',*,*,#7666,.F.);
#11308=ORIENTED_EDGE('',*,*,#7667,.F.);
#11309=ORIENTED_EDGE('',*,*,#7668,.F.);
#11310=ORIENTED_EDGE('',*,*,#7669,.F.);
#11311=ORIENTED_EDGE('',*,*,#7670,.F.);
#11312=ORIENTED_EDGE('',*,*,#7671,.F.);
#11313=ORIENTED_EDGE('',*,*,#7672,.F.);
#11314=ORIENTED_EDGE('',*,*,#7673,.F.);
#11315=ORIENTED_EDGE('',*,*,#7674,.F.);
#11316=ORIENTED_EDGE('',*,*,#7675,.F.);
#11317=ORIENTED_EDGE('',*,*,#7676,.F.);
#11318=ORIENTED_EDGE('',*,*,#7677,.F.);
#11319=ORIENTED_EDGE('',*,*,#7678,.F.);
#11320=ORIENTED_EDGE('',*,*,#7679,.F.);
#11321=ORIENTED_EDGE('',*,*,#7680,.F.);
#11322=ORIENTED_EDGE('',*,*,#7681,.F.);
#11323=ORIENTED_EDGE('',*,*,#7682,.T.);
#11324=ORIENTED_EDGE('',*,*,#7683,.T.);
#11325=ORIENTED_EDGE('',*,*,#7677,.T.);
#11326=ORIENTED_EDGE('',*,*,#7684,.T.);
#11327=ORIENTED_EDGE('',*,*,#7680,.T.);
#11328=ORIENTED_EDGE('',*,*,#7685,.T.);
#11329=ORIENTED_EDGE('',*,*,#7686,.T.);
#11330=ORIENTED_EDGE('',*,*,#7687,.T.);
#11331=ORIENTED_EDGE('',*,*,#7681,.T.);
#11332=ORIENTED_EDGE('',*,*,#7688,.T.);
#11333=ORIENTED_EDGE('',*,*,#7689,.T.);
#11334=ORIENTED_EDGE('',*,*,#7690,.T.);
#11335=ORIENTED_EDGE('',*,*,#7679,.T.);
#11336=ORIENTED_EDGE('',*,*,#7691,.T.);
#11337=ORIENTED_EDGE('',*,*,#7674,.T.);
#11338=ORIENTED_EDGE('',*,*,#7692,.T.);
#11339=ORIENTED_EDGE('',*,*,#7693,.T.);
#11340=ORIENTED_EDGE('',*,*,#7694,.T.);
#11341=ORIENTED_EDGE('',*,*,#7671,.T.);
#11342=ORIENTED_EDGE('',*,*,#7695,.T.);
#11343=ORIENTED_EDGE('',*,*,#7678,.T.);
#11344=ORIENTED_EDGE('',*,*,#7696,.T.);
#11345=ORIENTED_EDGE('',*,*,#7697,.T.);
#11346=ORIENTED_EDGE('',*,*,#7698,.T.);
#11347=ORIENTED_EDGE('',*,*,#7676,.T.);
#11348=ORIENTED_EDGE('',*,*,#7699,.T.);
#11349=ORIENTED_EDGE('',*,*,#7700,.T.);
#11350=ORIENTED_EDGE('',*,*,#7701,.T.);
#11351=ORIENTED_EDGE('',*,*,#7675,.T.);
#11352=ORIENTED_EDGE('',*,*,#7702,.T.);
#11353=ORIENTED_EDGE('',*,*,#7703,.T.);
#11354=ORIENTED_EDGE('',*,*,#7704,.T.);
#11355=ORIENTED_EDGE('',*,*,#7673,.T.);
#11356=ORIENTED_EDGE('',*,*,#7705,.T.);
#11357=ORIENTED_EDGE('',*,*,#7668,.T.);
#11358=ORIENTED_EDGE('',*,*,#7706,.T.);
#11359=ORIENTED_EDGE('',*,*,#7707,.T.);
#11360=ORIENTED_EDGE('',*,*,#7708,.T.);
#11361=ORIENTED_EDGE('',*,*,#7709,.T.);
#11362=ORIENTED_EDGE('',*,*,#7665,.T.);
#11363=ORIENTED_EDGE('',*,*,#7710,.T.);
#11364=ORIENTED_EDGE('',*,*,#7672,.T.);
#11365=ORIENTED_EDGE('',*,*,#7711,.T.);
#11366=ORIENTED_EDGE('',*,*,#7712,.T.);
#11367=ORIENTED_EDGE('',*,*,#7713,.T.);
#11368=ORIENTED_EDGE('',*,*,#7670,.T.);
#11369=ORIENTED_EDGE('',*,*,#7714,.T.);
#11370=ORIENTED_EDGE('',*,*,#7715,.T.);
#11371=ORIENTED_EDGE('',*,*,#7716,.T.);
#11372=ORIENTED_EDGE('',*,*,#7669,.T.);
#11373=ORIENTED_EDGE('',*,*,#7717,.T.);
#11374=ORIENTED_EDGE('',*,*,#7718,.T.);
#11375=ORIENTED_EDGE('',*,*,#7719,.T.);
#11376=ORIENTED_EDGE('',*,*,#7667,.T.);
#11377=ORIENTED_EDGE('',*,*,#7720,.T.);
#11378=ORIENTED_EDGE('',*,*,#7666,.T.);
#11379=ORIENTED_EDGE('',*,*,#7721,.T.);
#11380=ORIENTED_EDGE('',*,*,#7722,.T.);
#11381=ORIENTED_EDGE('',*,*,#7723,.T.);
#11382=ORIENTED_EDGE('',*,*,#7664,.T.);
#11383=ORIENTED_EDGE('',*,*,#7724,.T.);
#11384=ORIENTED_EDGE('',*,*,#7699,.F.);
#11385=ORIENTED_EDGE('',*,*,#7695,.F.);
#11386=ORIENTED_EDGE('',*,*,#7713,.F.);
#11387=ORIENTED_EDGE('',*,*,#7725,.T.);
#11388=ORIENTED_EDGE('',*,*,#7714,.F.);
#11389=ORIENTED_EDGE('',*,*,#7710,.F.);
#11390=ORIENTED_EDGE('',*,*,#7723,.F.);
#11391=ORIENTED_EDGE('',*,*,#7726,.T.);
#11392=ORIENTED_EDGE('',*,*,#7724,.F.);
#11393=ORIENTED_EDGE('',*,*,#7720,.F.);
#11394=ORIENTED_EDGE('',*,*,#7716,.F.);
#11395=ORIENTED_EDGE('',*,*,#7727,.T.);
#11396=ORIENTED_EDGE('',*,*,#7728,.F.);
#11397=ORIENTED_EDGE('',*,*,#7729,.T.);
#11398=ORIENTED_EDGE('',*,*,#7730,.F.);
#11399=ORIENTED_EDGE('',*,*,#7686,.F.);
#11400=ORIENTED_EDGE('',*,*,#7731,.F.);
#11401=ORIENTED_EDGE('',*,*,#7697,.F.);
#11402=ORIENTED_EDGE('',*,*,#7725,.F.);
#11403=ORIENTED_EDGE('',*,*,#7712,.F.);
#11404=ORIENTED_EDGE('',*,*,#7726,.F.);
#11405=ORIENTED_EDGE('',*,*,#7722,.F.);
#11406=ORIENTED_EDGE('',*,*,#7727,.F.);
#11407=ORIENTED_EDGE('',*,*,#7715,.F.);
#11408=ORIENTED_EDGE('',*,*,#7732,.F.);
#11409=ORIENTED_EDGE('',*,*,#7700,.F.);
#11410=ORIENTED_EDGE('',*,*,#7733,.F.);
#11411=ORIENTED_EDGE('',*,*,#7729,.F.);
#11412=ORIENTED_EDGE('',*,*,#7692,.F.);
#11413=ORIENTED_EDGE('',*,*,#7704,.F.);
#11414=ORIENTED_EDGE('',*,*,#7734,.F.);
#11415=ORIENTED_EDGE('',*,*,#7706,.F.);
#11416=ORIENTED_EDGE('',*,*,#7719,.F.);
#11417=ORIENTED_EDGE('',*,*,#7735,.F.);
#11418=ORIENTED_EDGE('',*,*,#7709,.F.);
#11419=ORIENTED_EDGE('',*,*,#7736,.F.);
#11420=ORIENTED_EDGE('',*,*,#7721,.F.);
#11421=ORIENTED_EDGE('',*,*,#7694,.F.);
#11422=ORIENTED_EDGE('',*,*,#7737,.F.);
#11423=ORIENTED_EDGE('',*,*,#7711,.F.);
#11424=ORIENTED_EDGE('',*,*,#7683,.F.);
#11425=ORIENTED_EDGE('',*,*,#7738,.F.);
#11426=ORIENTED_EDGE('',*,*,#7696,.F.);
#11427=ORIENTED_EDGE('',*,*,#7685,.F.);
#11428=ORIENTED_EDGE('',*,*,#7690,.F.);
#11429=ORIENTED_EDGE('',*,*,#7739,.F.);
#11430=ORIENTED_EDGE('',*,*,#7740,.T.);
#11431=ORIENTED_EDGE('',*,*,#7741,.T.);
#11432=ORIENTED_EDGE('',*,*,#7707,.F.);
#11433=ORIENTED_EDGE('',*,*,#7737,.T.);
#11434=ORIENTED_EDGE('',*,*,#7693,.F.);
#11435=ORIENTED_EDGE('',*,*,#7738,.T.);
#11436=ORIENTED_EDGE('',*,*,#7682,.F.);
#11437=ORIENTED_EDGE('',*,*,#7739,.T.);
#11438=ORIENTED_EDGE('',*,*,#7689,.F.);
#11439=ORIENTED_EDGE('',*,*,#7734,.T.);
#11440=ORIENTED_EDGE('',*,*,#7703,.F.);
#11441=ORIENTED_EDGE('',*,*,#7735,.T.);
#11442=ORIENTED_EDGE('',*,*,#7718,.F.);
#11443=ORIENTED_EDGE('',*,*,#7736,.T.);
#11444=ORIENTED_EDGE('',*,*,#7708,.F.);
#11445=ORIENTED_EDGE('',*,*,#7741,.F.);
#11446=ORIENTED_EDGE('',*,*,#7740,.F.);
#11447=ORIENTED_EDGE('',*,*,#7742,.F.);
#11448=ORIENTED_EDGE('',*,*,#7743,.T.);
#11449=ORIENTED_EDGE('',*,*,#7744,.T.);
#11450=ORIENTED_EDGE('',*,*,#7742,.T.);
#11451=ORIENTED_EDGE('',*,*,#7744,.F.);
#11452=ORIENTED_EDGE('',*,*,#7743,.F.);
#11453=ORIENTED_EDGE('',*,*,#7745,.T.);
#11454=ORIENTED_EDGE('',*,*,#7746,.F.);
#11455=ORIENTED_EDGE('',*,*,#7745,.F.);
#11456=ORIENTED_EDGE('',*,*,#7746,.T.);
#11457=ORIENTED_EDGE('',*,*,#7747,.T.);
#11458=ORIENTED_EDGE('',*,*,#7748,.T.);
#11459=ORIENTED_EDGE('',*,*,#7747,.F.);
#11460=ORIENTED_EDGE('',*,*,#7748,.F.);
#11461=ORIENTED_EDGE('',*,*,#7749,.T.);
#11462=ORIENTED_EDGE('',*,*,#7750,.F.);
#11463=ORIENTED_EDGE('',*,*,#7749,.F.);
#11464=ORIENTED_EDGE('',*,*,#7750,.T.);
#11465=ORIENTED_EDGE('',*,*,#7751,.T.);
#11466=ORIENTED_EDGE('',*,*,#7752,.T.);
#11467=ORIENTED_EDGE('',*,*,#7751,.F.);
#11468=ORIENTED_EDGE('',*,*,#7728,.T.);
#11469=ORIENTED_EDGE('',*,*,#7752,.F.);
#11470=ORIENTED_EDGE('',*,*,#7701,.F.);
#11471=ORIENTED_EDGE('',*,*,#7732,.T.);
#11472=ORIENTED_EDGE('',*,*,#7717,.F.);
#11473=ORIENTED_EDGE('',*,*,#7705,.F.);
#11474=ORIENTED_EDGE('',*,*,#7687,.F.);
#11475=ORIENTED_EDGE('',*,*,#7730,.T.);
#11476=ORIENTED_EDGE('',*,*,#7733,.T.);
#11477=ORIENTED_EDGE('',*,*,#7702,.F.);
#11478=ORIENTED_EDGE('',*,*,#7691,.F.);
#11479=ORIENTED_EDGE('',*,*,#7698,.F.);
#11480=ORIENTED_EDGE('',*,*,#7731,.T.);
#11481=ORIENTED_EDGE('',*,*,#7688,.F.);
#11482=ORIENTED_EDGE('',*,*,#7684,.F.);
#11766=PLANE('',#13536);
#11767=PLANE('',#13537);
#11768=PLANE('',#13538);
#11769=PLANE('',#13539);
#11770=PLANE('',#13540);
#11771=PLANE('',#13541);
#11772=PLANE('',#13542);
#11773=PLANE('',#13543);
#11774=PLANE('',#13544);
#11775=PLANE('',#13545);
#11776=PLANE('',#13546);
#11777=PLANE('',#13547);
#11778=PLANE('',#13548);
#11779=PLANE('',#13549);
#11780=PLANE('',#13550);
#11781=PLANE('',#13567);
#11782=PLANE('',#13579);
#11783=PLANE('',#13580);
#11784=PLANE('',#13581);
#11785=PLANE('',#13582);
#12441=ADVANCED_FACE('',(#2474),#11766,.T.);
#12442=ADVANCED_FACE('',(#2475),#11767,.T.);
#12443=ADVANCED_FACE('',(#2476),#11768,.T.);
#12444=ADVANCED_FACE('',(#2477),#11769,.T.);
#12445=ADVANCED_FACE('',(#2478),#11770,.T.);
#12446=ADVANCED_FACE('',(#2479),#11771,.T.);
#12447=ADVANCED_FACE('',(#2480),#1334,.T.);
#12448=ADVANCED_FACE('',(#2481),#11772,.T.);
#12449=ADVANCED_FACE('',(#2482),#1335,.T.);
#12450=ADVANCED_FACE('',(#2483),#1336,.T.);
#12451=ADVANCED_FACE('',(#2484),#11773,.T.);
#12452=ADVANCED_FACE('',(#2485),#11774,.T.);
#12453=ADVANCED_FACE('',(#2486),#1337,.T.);
#12454=ADVANCED_FACE('',(#2487),#1338,.T.);
#12455=ADVANCED_FACE('',(#2488),#11775,.T.);
#12456=ADVANCED_FACE('',(#2489),#11776,.T.);
#12457=ADVANCED_FACE('',(#2490),#1339,.T.);
#12458=ADVANCED_FACE('',(#2491),#11777,.T.);
#12459=ADVANCED_FACE('',(#2492),#11778,.T.);
#12460=ADVANCED_FACE('',(#2493),#11779,.T.);
#12461=ADVANCED_FACE('',(#2494),#11780,.T.);
#12462=ADVANCED_FACE('',(#2495),#445,.T.);
#12463=ADVANCED_FACE('',(#2496),#446,.T.);
#12464=ADVANCED_FACE('',(#2497),#447,.T.);
#12465=ADVANCED_FACE('',(#2498),#448,.T.);
#12466=ADVANCED_FACE('',(#2499),#449,.T.);
#12467=ADVANCED_FACE('',(#2500),#450,.T.);
#12468=ADVANCED_FACE('',(#2501),#451,.T.);
#12469=ADVANCED_FACE('',(#2502),#452,.T.);
#12470=ADVANCED_FACE('',(#2503,#1403),#11781,.T.);
#12471=ADVANCED_FACE('',(#2504),#453,.F.);
#12472=ADVANCED_FACE('',(#2505),#454,.F.);
#12473=ADVANCED_FACE('',(#2506),#455,.F.);
#12474=ADVANCED_FACE('',(#2507),#361,.F.);
#12475=ADVANCED_FACE('',(#2508),#456,.F.);
#12476=ADVANCED_FACE('',(#2509,#1404),#11782,.F.);
#12477=ADVANCED_FACE('',(#2510),#11783,.T.);
#12478=ADVANCED_FACE('',(#2511),#11784,.T.);
#12479=ADVANCED_FACE('',(#2512),#11785,.T.);
#12490=CLOSED_SHELL('',(#12441,#12442,#12443,#12444,#12445,#12446,#12447,
#12448,#12449,#12450,#12451,#12452,#12453,#12454,#12455,#12456,#12457,#12458,
#12459,#12460,#12461,#12462,#12463,#12464,#12465,#12466,#12467,#12468,#12469,
#12470,#12471,#12472,#12473,#12474,#12475,#12476,#12477,#12478,#12479));
#13535=AXIS2_PLACEMENT_3D('',#30988,#16144,#16145);
#13536=AXIS2_PLACEMENT_3D('',#30989,#16146,#16147);
#13537=AXIS2_PLACEMENT_3D('',#31006,#16149,#16150);
#13538=AXIS2_PLACEMENT_3D('',#31023,#16152,#16153);
#13539=AXIS2_PLACEMENT_3D('',#31040,#16155,#16156);
#13540=AXIS2_PLACEMENT_3D('',#31057,#16158,#16159);
#13541=AXIS2_PLACEMENT_3D('',#31074,#16161,#16162);
#13542=AXIS2_PLACEMENT_3D('',#31151,#16164,#16165);
#13543=AXIS2_PLACEMENT_3D('',#31279,#16168,#16169);
#13544=AXIS2_PLACEMENT_3D('',#31287,#16172,#16173);
#13545=AXIS2_PLACEMENT_3D('',#31420,#16176,#16177);
#13546=AXIS2_PLACEMENT_3D('',#31428,#16180,#16181);
#13547=AXIS2_PLACEMENT_3D('',#31496,#16184,#16185);
#13548=AXIS2_PLACEMENT_3D('',#31504,#16188,#16189);
#13549=AXIS2_PLACEMENT_3D('',#31508,#16190,#16191);
#13550=AXIS2_PLACEMENT_3D('',#31512,#16192,#16193);
#13551=AXIS2_PLACEMENT_3D('',#31516,#16194,#16195);
#13552=AXIS2_PLACEMENT_3D('',#31518,#16196,#16197);
#13553=AXIS2_PLACEMENT_3D('',#31533,#16199,#16200);
#13554=AXIS2_PLACEMENT_3D('',#31534,#16201,#16202);
#13555=AXIS2_PLACEMENT_3D('',#31535,#16203,#16204);
#13556=AXIS2_PLACEMENT_3D('',#31536,#16205,#16206);
#13557=AXIS2_PLACEMENT_3D('',#31537,#16207,#16208);
#13558=AXIS2_PLACEMENT_3D('',#31538,#16209,#16210);
#13559=AXIS2_PLACEMENT_3D('',#31539,#16211,#16212);
#13560=AXIS2_PLACEMENT_3D('',#31540,#16213,#16214);
#13561=AXIS2_PLACEMENT_3D('',#31541,#16215,#16216);
#13562=AXIS2_PLACEMENT_3D('',#31542,#16217,#16218);
#13563=AXIS2_PLACEMENT_3D('',#31543,#16219,#16220);
#13564=AXIS2_PLACEMENT_3D('',#31544,#16221,#16222);
#13565=AXIS2_PLACEMENT_3D('',#31545,#16223,#16224);
#13566=AXIS2_PLACEMENT_3D('',#31547,#16225,#16226);
#13567=AXIS2_PLACEMENT_3D('',#31549,#16228,#16229);
#13568=AXIS2_PLACEMENT_3D('',#31551,#16230,#16231);
#13569=AXIS2_PLACEMENT_3D('',#31552,#16232,#16233);
#13570=AXIS2_PLACEMENT_3D('',#31554,#16234,#16235);
#13571=AXIS2_PLACEMENT_3D('',#31556,#16237,#16238);
#13572=AXIS2_PLACEMENT_3D('',#31559,#16240,#16241);
#13573=AXIS2_PLACEMENT_3D('',#31560,#16242,#16243);
#13574=AXIS2_PLACEMENT_3D('',#31563,#16245,#16246);
#13575=AXIS2_PLACEMENT_3D('',#31564,#16247,#16248);
#13576=AXIS2_PLACEMENT_3D('',#31567,#16250,#16251);
#13577=AXIS2_PLACEMENT_3D('',#31568,#16252,#16253);
#13578=AXIS2_PLACEMENT_3D('',#31571,#16255,#16256);
#13579=AXIS2_PLACEMENT_3D('',#31572,#16257,#16258);
#13580=AXIS2_PLACEMENT_3D('',#31573,#16259,#16260);
#13581=AXIS2_PLACEMENT_3D('',#31574,#16261,#16262);
#13582=AXIS2_PLACEMENT_3D('',#31575,#16263,#16264);
#16144=DIRECTION('axis',(0.,0.,1.));
#16145=DIRECTION('refdir',(1.,0.,0.));
#16146=DIRECTION('center_axis',(0.804732485689015,-0.464612517239211,0.369514323540269));
#16147=DIRECTION('ref_axis',(0.417287908209953,0.,-0.908774340340748));
#16148=DIRECTION('',(-0.499999999999997,-0.86602540378444,-6.10464344883671E-15));
#16149=DIRECTION('center_axis',(-8.89195164525175E-13,-0.929225034476892,
0.369514323540265));
#16150=DIRECTION('ref_axis',(0.,-0.369514323540265,-0.929225034476892));
#16151=DIRECTION('',(-1.,0.,-1.52616086220918E-15));
#16152=DIRECTION('center_axis',(0.804732485689902,0.464612517237679,0.369514323540264));
#16153=DIRECTION('ref_axis',(0.417287908209569,0.,-0.908774340340925));
#16154=DIRECTION('',(0.499999999999999,-0.866025403784439,-6.10464344883671E-15));
#16155=DIRECTION('center_axis',(-0.804732485689905,-0.464612517237674,0.369514323540265));
#16156=DIRECTION('ref_axis',(0.417287908209569,0.,0.908774340340924));
#16157=DIRECTION('',(-0.499999999999999,0.866025403784439,-3.05232172441835E-15));
#16158=DIRECTION('center_axis',(8.86349292865986E-13,0.92922503447689,0.369514323540268));
#16159=DIRECTION('ref_axis',(0.,-0.369514323540268,0.92922503447689));
#16160=DIRECTION('',(1.,3.05232172441836E-15,-4.57848258662754E-15));
#16161=DIRECTION('center_axis',(-0.804732485689018,0.464612517239214,0.369514323540261));
#16162=DIRECTION('ref_axis',(0.417287908209945,0.,0.908774340340752));
#16163=DIRECTION('',(0.499999999999999,0.866025403784439,-6.10464344883671E-15));
#16164=DIRECTION('center_axis',(-0.866025403784439,0.499999999999999,0.));
#16165=DIRECTION('ref_axis',(0.,0.,1.));
#16166=DIRECTION('',(0.,0.,1.));
#16167=DIRECTION('',(0.,0.,-1.));
#16168=DIRECTION('center_axis',(-3.05232172441836E-15,1.,0.));
#16169=DIRECTION('ref_axis',(0.,0.,1.));
#16170=DIRECTION('',(0.,0.,1.));
#16171=DIRECTION('',(0.,0.,-1.));
#16172=DIRECTION('center_axis',(-0.866025403784439,-0.499999999999999,0.));
#16173=DIRECTION('ref_axis',(0.,0.,1.));
#16174=DIRECTION('',(0.,0.,1.));
#16175=DIRECTION('',(0.,0.,-1.));
#16176=DIRECTION('center_axis',(0.866025403784439,0.499999999999999,0.));
#16177=DIRECTION('ref_axis',(0.,0.,-1.));
#16178=DIRECTION('',(0.,0.,1.));
#16179=DIRECTION('',(0.,0.,-1.));
#16180=DIRECTION('center_axis',(0.,-1.,0.));
#16181=DIRECTION('ref_axis',(0.,0.,-1.));
#16182=DIRECTION('',(0.,0.,1.));
#16183=DIRECTION('',(0.,0.,-1.));
#16184=DIRECTION('center_axis',(0.86602540378444,-0.499999999999997,0.));
#16185=DIRECTION('ref_axis',(0.,0.,-1.));
#16186=DIRECTION('',(0.,0.,1.));
#16187=DIRECTION('',(0.,0.,-1.));
#16188=DIRECTION('center_axis',(0.5,0.866025403784439,0.));
#16189=DIRECTION('ref_axis',(-0.866025403784439,0.5,0.));
#16190=DIRECTION('center_axis',(1.,-3.84592537276713E-16,0.));
#16191=DIRECTION('ref_axis',(3.84592537276713E-16,1.,0.));
#16192=DIRECTION('center_axis',(0.5,-0.866025403784439,0.));
#16193=DIRECTION('ref_axis',(0.866025403784439,0.5,0.));
#16194=DIRECTION('center_axis',(0.,0.,1.));
#16195=DIRECTION('ref_axis',(1.,0.,0.));
#16196=DIRECTION('center_axis',(0.,0.,-1.));
#16197=DIRECTION('ref_axis',(1.,0.,0.));
#16198=DIRECTION('',(-0.866025403784439,-1.06057523872491E-16,0.5));
#16199=DIRECTION('center_axis',(0.,0.,-1.));
#16200=DIRECTION('ref_axis',(1.,0.,0.));
#16201=DIRECTION('center_axis',(0.,0.,1.));
#16202=DIRECTION('ref_axis',(-1.,-6.12323399573677E-17,0.));
#16203=DIRECTION('center_axis',(0.,0.,-1.));
#16204=DIRECTION('ref_axis',(1.,0.,0.));
#16205=DIRECTION('center_axis',(0.,0.,1.));
#16206=DIRECTION('ref_axis',(-1.,-6.12323399573677E-17,0.));
#16207=DIRECTION('center_axis',(0.,0.,-1.));
#16208=DIRECTION('ref_axis',(1.,0.,0.));
#16209=DIRECTION('center_axis',(0.,0.,1.));
#16210=DIRECTION('ref_axis',(-1.,-6.12323399573677E-17,0.));
#16211=DIRECTION('center_axis',(0.,0.,-1.));
#16212=DIRECTION('ref_axis',(1.,0.,0.));
#16213=DIRECTION('center_axis',(0.,0.,1.));
#16214=DIRECTION('ref_axis',(-1.,-6.12323399573677E-17,0.));
#16215=DIRECTION('center_axis',(0.,0.,-1.));
#16216=DIRECTION('ref_axis',(1.,0.,0.));
#16217=DIRECTION('center_axis',(0.,0.,1.));
#16218=DIRECTION('ref_axis',(-1.,-6.12323399573677E-17,0.));
#16219=DIRECTION('center_axis',(0.,0.,-1.));
#16220=DIRECTION('ref_axis',(1.,0.,0.));
#16221=DIRECTION('center_axis',(0.,0.,1.));
#16222=DIRECTION('ref_axis',(-1.,-6.12323399573677E-17,0.));
#16223=DIRECTION('center_axis',(0.,-2.87609195051533E-15,-1.));
#16224=DIRECTION('ref_axis',(-1.,-3.18828070427431E-17,0.));
#16225=DIRECTION('center_axis',(0.,0.,-1.));
#16226=DIRECTION('ref_axis',(-1.,0.,0.));
#16227=DIRECTION('',(0.965925826289069,-5.95299148384376E-16,-0.25881904510252));
#16228=DIRECTION('center_axis',(0.,0.,1.));
#16229=DIRECTION('ref_axis',(1.,0.,0.));
#16230=DIRECTION('center_axis',(0.,0.,1.));
#16231=DIRECTION('ref_axis',(1.,0.,0.));
#16232=DIRECTION('center_axis',(0.,1.36140975242952E-15,1.));
#16233=DIRECTION('ref_axis',(1.,2.90395481232862E-17,0.));
#16234=DIRECTION('center_axis',(0.,0.,-1.));
#16235=DIRECTION('ref_axis',(1.,6.12323399573676E-17,0.));
#16236=DIRECTION('',(-0.923879532511287,6.07302523999323E-16,0.382683432365089));
#16237=DIRECTION('center_axis',(0.,0.,1.));
#16238=DIRECTION('ref_axis',(1.,0.,0.));
#16239=DIRECTION('',(0.707106781186547,8.65956056235493E-17,-0.707106781186548));
#16240=DIRECTION('center_axis',(0.,0.,1.));
#16241=DIRECTION('ref_axis',(1.,6.12323399573676E-17,0.));
#16242=DIRECTION('center_axis',(0.,-5.46318868466739E-16,1.));
#16243=DIRECTION('ref_axis',(1.,3.13437485667187E-17,0.));
#16244=DIRECTION('',(0.382683432365089,5.63592758139109E-16,-0.923879532511287));
#16245=DIRECTION('center_axis',(0.,0.,-1.));
#16246=DIRECTION('ref_axis',(1.,0.,0.));
#16247=DIRECTION('center_axis',(0.,0.,1.));
#16248=DIRECTION('ref_axis',(1.,0.,0.));
#16249=DIRECTION('',(0.,0.,-1.));
#16250=DIRECTION('center_axis',(0.,0.,1.));
#16251=DIRECTION('ref_axis',(1.,0.,0.));
#16252=DIRECTION('center_axis',(0.,0.,-1.));
#16253=DIRECTION('ref_axis',(1.,0.,0.));
#16254=DIRECTION('',(-0.707106781186547,-8.65956056235493E-17,-0.707106781186548));
#16255=DIRECTION('center_axis',(0.,0.,-1.));
#16256=DIRECTION('ref_axis',(1.,0.,0.));
#16257=DIRECTION('center_axis',(0.,0.,1.));
#16258=DIRECTION('ref_axis',(1.,0.,0.));
#16259=DIRECTION('center_axis',(-0.5,-0.866025403784439,0.));
#16260=DIRECTION('ref_axis',(0.866025403784439,-0.5,0.));
#16261=DIRECTION('center_axis',(-1.,-1.92296268638356E-16,0.));
#16262=DIRECTION('ref_axis',(1.92296268638356E-16,-1.,0.));
#16263=DIRECTION('center_axis',(-0.5,0.866025403784439,0.));
#16264=DIRECTION('ref_axis',(-0.866025403784439,-0.5,0.));
#30988=CARTESIAN_POINT('',(0.,0.,0.));
#30989=CARTESIAN_POINT('Origin',(0.5,-0.267675134594871,0.445023951189801));
#30990=CARTESIAN_POINT('',(0.5,-0.267675134594871,0.445023951189801));
#30991=CARTESIAN_POINT('',(0.481813466520527,-0.299175134594813,0.445023951189787));
#30992=CARTESIAN_POINT('',(0.5,-0.267675134594813,0.445023951189788));
#30993=CARTESIAN_POINT('',(0.481096510297973,-0.277761199726725,0.473510370999757));
#30994=CARTESIAN_POINT('Ctrl Pts',(0.5,-0.267675134594871,0.445023951189802));
#30995=CARTESIAN_POINT('Ctrl Pts',(0.496851093414489,-0.269349908597711,
0.449775881890813));
#30996=CARTESIAN_POINT('Ctrl Pts',(0.493701109562143,-0.271027926795793,
0.454526079554539));
#30997=CARTESIAN_POINT('Ctrl Pts',(0.487399980032294,-0.274389929231452,
0.464021503658784));
#30998=CARTESIAN_POINT('Ctrl Pts',(0.484248729970766,-0.276073967840828,
0.468766889063092));
#30999=CARTESIAN_POINT('Ctrl Pts',(0.481096510297973,-0.277761199726724,
0.473510370999757));
#31000=CARTESIAN_POINT('Ctrl Pts',(0.481096510297973,-0.277761199726725,
0.473510370999757));
#31001=CARTESIAN_POINT('Ctrl Pts',(0.481211435993815,-0.281334765706086,
0.468766825717716));
#31002=CARTESIAN_POINT('Ctrl Pts',(0.481328642403551,-0.284905895274937,
0.46402137691612));
#31003=CARTESIAN_POINT('Ctrl Pts',(0.481567627773124,-0.292043834604859,
0.454525952714809));
#31004=CARTESIAN_POINT('Ctrl Pts',(0.481689411716076,-0.295610762084322,
0.449775818448415));
#31005=CARTESIAN_POINT('Ctrl Pts',(0.4818134665205,-0.299175134594829,0.445023951189826));
#31006=CARTESIAN_POINT('Origin',(3.40159364172662E-17,-0.555522399453449,
0.473510370999757));
#31007=CARTESIAN_POINT('',(3.40159364172662E-17,-0.555522399453449,0.473510370999757));
#31008=CARTESIAN_POINT('',(0.0181865334794225,-0.566850269189655,0.445023951189802));
#31009=CARTESIAN_POINT('Ctrl Pts',(0.0181865334794225,-0.566850269189655,
0.445023951189802));
#31010=CARTESIAN_POINT('Ctrl Pts',(0.0151616833547915,-0.564960623093991,
0.449775881890529));
#31011=CARTESIAN_POINT('Ctrl Pts',(0.0121334850409848,-0.563071666155339,
0.454526079554383));
#31012=CARTESIAN_POINT('Ctrl Pts',(0.00607134075855177,-0.559295729127382,
0.464021503659636));
#31013=CARTESIAN_POINT('Ctrl Pts',(0.00303729551137823,-0.557408685825276,
0.468766889063527));
#31014=CARTESIAN_POINT('Ctrl Pts',(-3.36036318723674E-16,-0.555522399453449,
0.473510370999756));
#31015=CARTESIAN_POINT('',(-0.0181865334794733,-0.566850269189626,0.445023951189787));
#31016=CARTESIAN_POINT('Ctrl Pts',(-2.12685567010027E-16,-0.555522399453449,
0.473510370999756));
#31017=CARTESIAN_POINT('Ctrl Pts',(-0.00303733607236141,-0.557408711015311,
0.468766825717629));
#31018=CARTESIAN_POINT('Ctrl Pts',(-0.00607142179437835,-0.559295779528088,
0.464021376915948));
#31019=CARTESIAN_POINT('Ctrl Pts',(-0.0121335658997963,-0.56307171659412,
0.454525952714919));
#31020=CARTESIAN_POINT('Ctrl Pts',(-0.015161723738915,-0.564960648322172,
0.449775818448647));
#31021=CARTESIAN_POINT('Ctrl Pts',(-0.0181865334794998,-0.56685026918961,
0.445023951189826));
#31022=CARTESIAN_POINT('',(0.018186533479473,-0.566850269189626,0.445023951189787));
#31023=CARTESIAN_POINT('Origin',(0.481813466520577,0.299175134594784,0.445023951189801));
#31024=CARTESIAN_POINT('',(0.481813466520577,0.299175134594784,0.445023951189801));
#31025=CARTESIAN_POINT('',(0.5,0.267675134594813,0.445023951189787));
#31026=CARTESIAN_POINT('',(0.481813466520527,0.299175134594813,0.445023951189788));
#31027=CARTESIAN_POINT('',(0.481096510297973,0.277761199726725,0.473510370999757));
#31028=CARTESIAN_POINT('Ctrl Pts',(0.481813466520577,0.299175134594784,
0.445023951189802));
#31029=CARTESIAN_POINT('Ctrl Pts',(0.481689410059888,0.295610714496447,
0.449775881890441));
#31030=CARTESIAN_POINT('Ctrl Pts',(0.481567624521262,0.292043739359626,
0.45452607955435));
#31031=CARTESIAN_POINT('Ctrl Pts',(0.48132863927319,0.284905799896003,0.464021503659138));
#31032=CARTESIAN_POINT('Ctrl Pts',(0.481211434459105,0.281334717984484,
0.468766889063272));
#31033=CARTESIAN_POINT('Ctrl Pts',(0.481096510297974,0.277761199726724,
0.473510370999757));
#31034=CARTESIAN_POINT('Ctrl Pts',(0.481096510297974,0.277761199726724,
0.473510370999757));
#31035=CARTESIAN_POINT('Ctrl Pts',(0.484248772066078,0.276073945309214,
0.46876682571778));
#31036=CARTESIAN_POINT('Ctrl Pts',(0.487400064197721,0.274389884253135,
0.464021376916268));
#31037=CARTESIAN_POINT('Ctrl Pts',(0.493701193672944,0.271027881989329,
0.454525952714879));
#31038=CARTESIAN_POINT('Ctrl Pts',(0.496851135455045,0.269349886237992,
0.449775818448557));
#31039=CARTESIAN_POINT('Ctrl Pts',(0.5,0.267675134594782,0.445023951189826));
#31040=CARTESIAN_POINT('Origin',(-0.481096510297974,-0.277761199726724,
0.473510370999757));
#31041=CARTESIAN_POINT('',(-0.481096510297974,-0.277761199726724,0.473510370999757));
#31042=CARTESIAN_POINT('',(-0.481813466520577,-0.299175134594784,0.445023951189802));
#31043=CARTESIAN_POINT('Ctrl Pts',(-0.481813466520578,-0.299175134594784,
0.445023951189801));
#31044=CARTESIAN_POINT('Ctrl Pts',(-0.481689410059868,-0.295610714495857,
0.449775881891228));
#31045=CARTESIAN_POINT('Ctrl Pts',(-0.481567624521253,-0.292043739359335,
0.454526079554737));
#31046=CARTESIAN_POINT('Ctrl Pts',(-0.481328639273198,-0.284905799896236,
0.464021503658828));
#31047=CARTESIAN_POINT('Ctrl Pts',(-0.481211434459109,-0.281334717984605,
0.468766889063111));
#31048=CARTESIAN_POINT('Ctrl Pts',(-0.481096510297974,-0.277761199726725,
0.473510370999757));
#31049=CARTESIAN_POINT('',(-0.5,-0.267675134594813,0.445023951189787));
#31050=CARTESIAN_POINT('Ctrl Pts',(-0.481096510297974,-0.277761199726724,
0.473510370999757));
#31051=CARTESIAN_POINT('Ctrl Pts',(-0.484248772066081,-0.276073945309212,
0.468766825717777));
#31052=CARTESIAN_POINT('Ctrl Pts',(-0.487400064197745,-0.274389884253123,
0.464021376916233));
#31053=CARTESIAN_POINT('Ctrl Pts',(-0.493701193672965,-0.271027881989318,
0.454525952714847));
#31054=CARTESIAN_POINT('Ctrl Pts',(-0.496851135455069,-0.269349886237979,
0.44977581844852));
#31055=CARTESIAN_POINT('Ctrl Pts',(-0.5,-0.267675134594782,0.445023951189826));
#31056=CARTESIAN_POINT('',(-0.481813466520527,-0.299175134594813,0.445023951189787));
#31057=CARTESIAN_POINT('Origin',(-0.0181865334794227,0.566850269189655,
0.445023951189802));
#31058=CARTESIAN_POINT('',(-0.0181865334794227,0.566850269189655,0.445023951189802));
#31059=CARTESIAN_POINT('',(0.0181865334794732,0.566850269189626,0.445023951189787));
#31060=CARTESIAN_POINT('',(-0.0181865334794732,0.566850269189626,0.445023951189788));
#31061=CARTESIAN_POINT('',(3.40159364172662E-17,0.555522399453449,0.473510370999757));
#31062=CARTESIAN_POINT('Ctrl Pts',(-0.0181865334794227,0.566850269189655,
0.445023951189802));
#31063=CARTESIAN_POINT('Ctrl Pts',(-0.0151616833546625,0.564960623093911,
0.449775881890732));
#31064=CARTESIAN_POINT('Ctrl Pts',(-0.0121334850409241,0.563071666155301,
0.454526079554478));
#31065=CARTESIAN_POINT('Ctrl Pts',(-0.00607134075884239,0.559295729127563,
0.464021503659181));
#31066=CARTESIAN_POINT('Ctrl Pts',(-0.00303729551152701,0.557408685825368,
0.468766889063295));
#31067=CARTESIAN_POINT('Ctrl Pts',(-2.12685567010027E-16,0.555522399453449,
0.473510370999757));
#31068=CARTESIAN_POINT('Ctrl Pts',(1.57366688130913E-16,0.555522399453449,
0.473510370999757));
#31069=CARTESIAN_POINT('Ctrl Pts',(0.00303733607213158,0.557408711015168,
0.468766825717988));
#31070=CARTESIAN_POINT('Ctrl Pts',(0.00607142179389414,0.559295779527786,
0.464021376916707));
#31071=CARTESIAN_POINT('Ctrl Pts',(0.012133565899859,0.563071716594158,
0.454525952714821));
#31072=CARTESIAN_POINT('Ctrl Pts',(0.015161723739062,0.564960648322264,
0.449775818448416));
#31073=CARTESIAN_POINT('Ctrl Pts',(0.0181865334794999,0.56685026918961,
0.445023951189826));
#31074=CARTESIAN_POINT('Origin',(-0.481096510297974,0.277761199726725,0.473510370999757));
#31075=CARTESIAN_POINT('',(-0.481096510297974,0.277761199726725,0.473510370999757));
#31076=CARTESIAN_POINT('',(-0.5,0.267675134594871,0.445023951189801));
#31077=CARTESIAN_POINT('Ctrl Pts',(-0.5,0.267675134594871,0.445023951189802));
#31078=CARTESIAN_POINT('Ctrl Pts',(-0.496851093414684,0.269349908597607,
0.44977588189052));
#31079=CARTESIAN_POINT('Ctrl Pts',(-0.493701109562242,0.271027926795741,
0.45452607955439));
#31080=CARTESIAN_POINT('Ctrl Pts',(-0.487399980032028,0.274389929231594,
0.464021503659185));
#31081=CARTESIAN_POINT('Ctrl Pts',(-0.484248729970629,0.276073967840903,
0.468766889063299));
#31082=CARTESIAN_POINT('Ctrl Pts',(-0.481096510297974,0.277761199726725,
0.473510370999757));
#31083=CARTESIAN_POINT('',(-0.481813466520527,0.299175134594813,0.445023951189787));
#31084=CARTESIAN_POINT('Ctrl Pts',(-0.481096510297974,0.277761199726724,
0.473510370999757));
#31085=CARTESIAN_POINT('Ctrl Pts',(-0.481211435993815,0.281334765706079,
0.468766825717724));
#31086=CARTESIAN_POINT('Ctrl Pts',(-0.48132864240355,0.284905895274894,
0.464021376916177));
#31087=CARTESIAN_POINT('Ctrl Pts',(-0.48156762777312,0.292043834604734,
0.454525952714975));
#31088=CARTESIAN_POINT('Ctrl Pts',(-0.481689411716068,0.295610762084098,
0.449775818448714));
#31089=CARTESIAN_POINT('Ctrl Pts',(-0.4818134665205,0.299175134594828,0.445023951189826));
#31090=CARTESIAN_POINT('',(-0.5,0.267675134594813,0.445023951189788));
#31091=CARTESIAN_POINT('Ctrl Pts',(-0.483544441026001,0.298175755998117,
0.444468924013264));
#31092=CARTESIAN_POINT('Ctrl Pts',(-0.406912985802199,0.342418947299972,
0.469110141953084));
#31093=CARTESIAN_POINT('Ctrl Pts',(-0.257908341391985,0.428446818860713,
0.495972649874704));
#31094=CARTESIAN_POINT('Ctrl Pts',(-0.118630832605733,0.508858726050516,
0.477323881266358));
#31095=CARTESIAN_POINT('Ctrl Pts',(-0.0164555589739993,0.567849647786322,
0.444468924013264));
#31096=CARTESIAN_POINT('Ctrl Pts',(-0.482728464116659,0.291370903907653,
0.454149406342095));
#31097=CARTESIAN_POINT('Ctrl Pts',(-0.405668349322323,0.335995410650277,
0.479195744603699));
#31098=CARTESIAN_POINT('Ctrl Pts',(-0.255104666887408,0.42318499384238,
0.506818674741199));
#31099=CARTESIAN_POINT('Ctrl Pts',(-0.113871724472838,0.504508880129862,
0.487544524024234));
#31100=CARTESIAN_POINT('Ctrl Pts',(-0.0109703726493329,0.563740565008697,
0.454149406342095));
#31101=CARTESIAN_POINT('Ctrl Pts',(-0.481912487207316,0.284566051817189,
0.463829888670926));
#31102=CARTESIAN_POINT('Ctrl Pts',(-0.404423712842447,0.329571874000582,
0.489281347254314));
#31103=CARTESIAN_POINT('Ctrl Pts',(-0.252300992382831,0.417923168824047,
0.517664699607693));
#31104=CARTESIAN_POINT('Ctrl Pts',(-0.109112616339942,0.500159034209207,
0.49776516678211));
#31105=CARTESIAN_POINT('Ctrl Pts',(-0.00548518632466643,0.559631482231073,
0.463829888670926));
#31106=CARTESIAN_POINT('Ctrl Pts',(-0.481096510297974,0.277761199726724,
0.473510370999756));
#31107=CARTESIAN_POINT('Ctrl Pts',(-0.403179076362571,0.323148337350887,
0.499366949904929));
#31108=CARTESIAN_POINT('Ctrl Pts',(-0.249497317878254,0.412661343805713,
0.528510724474188));
#31109=CARTESIAN_POINT('Ctrl Pts',(-0.104353508207047,0.495809188288553,
0.507985809539986));
#31110=CARTESIAN_POINT('Ctrl Pts',(1.38777878078145E-17,0.555522399453449,
0.473510370999757));
#31111=CARTESIAN_POINT('',(-0.332273583321365,0.364361108482639,0.50952199081629));
#31112=CARTESIAN_POINT('',(-0.149406387802791,0.469927086065252,0.50977488582138));
#31113=CARTESIAN_POINT('Ctrl Pts',(-0.332255993860912,0.364371421655621,
0.509523338656206));
#31114=CARTESIAN_POINT('Ctrl Pts',(-0.318279946918584,0.373351253352375,
0.510249567790552));
#31115=CARTESIAN_POINT('Ctrl Pts',(-0.304245988201247,0.38215746972964,
0.510799578547925));
#31116=CARTESIAN_POINT('Ctrl Pts',(-0.290111717192355,0.390806403397501,
0.511195921402465));
#31117=CARTESIAN_POINT('Ctrl Pts',(-0.287860051912662,0.392184224979812,
0.511259060947749));
#31118=CARTESIAN_POINT('Ctrl Pts',(-0.28560575614068,0.393558099738657,
0.511318349002632));
#31119=CARTESIAN_POINT('Ctrl Pts',(-0.283348567387494,0.394928140744563,
0.511373928077867));
#31120=CARTESIAN_POINT('Ctrl Pts',(-0.280216737305738,0.39682906091771,
0.511451043569202));
#31121=CARTESIAN_POINT('Ctrl Pts',(-0.277081273935527,0.398721437766428,
0.511520951504384));
#31122=CARTESIAN_POINT('Ctrl Pts',(-0.273941641913879,0.400605537752242,
0.511584044834106));
#31123=CARTESIAN_POINT('Ctrl Pts',(-0.267927330155416,0.404214739283079,
0.511704907072805));
#31124=CARTESIAN_POINT('Ctrl Pts',(-0.261897755700511,0.407793556450529,
0.511800747922412));
#31125=CARTESIAN_POINT('Ctrl Pts',(-0.25584883066306,0.411344203910499,
0.511868640474087));
#31126=CARTESIAN_POINT('Ctrl Pts',(-0.248348767769815,0.415746652130082,
0.511952820457207));
#31127=CARTESIAN_POINT('Ctrl Pts',(-0.240826093245991,0.420101623101484,
0.511993883112242));
#31128=CARTESIAN_POINT('Ctrl Pts',(-0.233273179007016,0.424413640109889,
0.511986957182662));
#31129=CARTESIAN_POINT('Ctrl Pts',(-0.224651569134181,0.429335783700459,
0.511979051272312));
#31130=CARTESIAN_POINT('Ctrl Pts',(-0.215999456170061,0.434196874243185,
0.511908560978455));
#31131=CARTESIAN_POINT('Ctrl Pts',(-0.207306027932602,0.439003856133907,
0.511770158465883));
#31132=CARTESIAN_POINT('Ctrl Pts',(-0.192599818167039,0.44713557150479,
0.511536030303048));
#31133=CARTESIAN_POINT('Ctrl Pts',(-0.17781016961573,0.455093185534583,
0.511107142930621));
#31134=CARTESIAN_POINT('Ctrl Pts',(-0.162894469075894,0.462908436068343,
0.51047380092448));
#31135=CARTESIAN_POINT('Ctrl Pts',(-0.15843407026544,0.465245512633475,
0.510284406003118));
#31136=CARTESIAN_POINT('Ctrl Pts',(-0.153964937425956,0.467568528701837,
0.51007694825866));
#31137=CARTESIAN_POINT('Ctrl Pts',(-0.149486235114875,0.469878234401755,
0.509851518489547));
#31138=CARTESIAN_POINT('Ctrl Pts',(-0.149486235113333,0.46987823440264,
0.50985151848933));
#31139=CARTESIAN_POINT('Ctrl Pts',(-0.10320209198028,0.496453452351216,
0.503326883310332));
#31140=CARTESIAN_POINT('Ctrl Pts',(-0.0545240825613662,0.524322604530414,
0.491523580997232));
#31141=CARTESIAN_POINT('Ctrl Pts',(1.38777878078145E-17,0.555522399453449,
0.473510370999757));
#31142=CARTESIAN_POINT('Ctrl Pts',(-0.0181867260015379,0.56685015803696,
0.44502415632149));
#31143=CARTESIAN_POINT('Ctrl Pts',(-0.119531026231089,0.508338999018595,
0.47744392523402));
#31144=CARTESIAN_POINT('Ctrl Pts',(-0.257939671025404,0.428428730688425,
0.495826064932766));
#31145=CARTESIAN_POINT('Ctrl Pts',(-0.405950132909958,0.342974850676497,
0.469283267869301));
#31146=CARTESIAN_POINT('Ctrl Pts',(-0.48181328528966,0.299175239228503,
0.445024047543947));
#31147=CARTESIAN_POINT('Ctrl Pts',(-0.481096510297974,0.277761199726724,
0.473510370999756));
#31148=CARTESIAN_POINT('Ctrl Pts',(-0.426814654021077,0.309380542881391,
0.491523580997232));
#31149=CARTESIAN_POINT('Ctrl Pts',(-0.378382919626527,0.337590700753812,
0.503049636797564));
#31150=CARTESIAN_POINT('Ctrl Pts',(-0.332255993862453,0.364371421654726,
0.50952333865599));
#31151=CARTESIAN_POINT('Origin',(-0.490906733260264,0.283425134594813,0.));
#31152=CARTESIAN_POINT('',(-0.481813466520527,0.299175134594813,0.0531981726275096));
#31153=CARTESIAN_POINT('',(-0.5,0.267675134594813,0.0531981726275097));
#31154=CARTESIAN_POINT('Ctrl Pts',(-0.481813466520527,0.299175134594813,
0.0531981726275096));
#31155=CARTESIAN_POINT('Ctrl Pts',(-0.490906733260264,0.283425134594813,
0.0528614692578827));
#31156=CARTESIAN_POINT('Ctrl Pts',(-0.5,0.267675134594813,0.0531981726275097));
#31157=CARTESIAN_POINT('',(-0.5,0.267675134594813,0.));
#31158=CARTESIAN_POINT('',(-0.481813466520527,0.299175134594813,0.));
#31159=CARTESIAN_POINT('Ctrl Pts',(-0.5,-0.269673891788205,0.444468924013264));
#31160=CARTESIAN_POINT('Ctrl Pts',(-0.5,-0.181187509184495,0.469110141953084));
#31161=CARTESIAN_POINT('Ctrl Pts',(-0.5,-0.00912777933363359,0.495992583115463));
#31162=CARTESIAN_POINT('Ctrl Pts',(-0.5,0.151692048316594,0.477323881266358));
#31163=CARTESIAN_POINT('Ctrl Pts',(-0.5,0.269673891788205,0.444468924013264));
#31164=CARTESIAN_POINT('Ctrl Pts',(-0.493698836765991,-0.272369661101045,
0.454149406342095));
#31165=CARTESIAN_POINT('Ctrl Pts',(-0.493814735839286,-0.183321390699293,
0.479195744603699));
#31166=CARTESIAN_POINT('Ctrl Pts',(-0.494041168132572,-0.00933048749449408,
0.506838267803536));
#31167=CARTESIAN_POINT('Ctrl Pts',(-0.493853368863718,0.153638633898712,
0.487544524024234));
#31168=CARTESIAN_POINT('Ctrl Pts',(-0.493698836765991,0.272369661101045,
0.454149406342095));
#31169=CARTESIAN_POINT('Ctrl Pts',(-0.487397673531982,-0.275065430413885,
0.463829888670926));
#31170=CARTESIAN_POINT('Ctrl Pts',(-0.487629471678572,-0.185455272214091,
0.489281347254314));
#31171=CARTESIAN_POINT('Ctrl Pts',(-0.488082336265144,-0.00953319565535434,
0.517683952491609));
#31172=CARTESIAN_POINT('Ctrl Pts',(-0.487706737727435,0.155585219480829,
0.49776516678211));
#31173=CARTESIAN_POINT('Ctrl Pts',(-0.487397673531982,0.275065430413885,
0.463829888670926));
#31174=CARTESIAN_POINT('Ctrl Pts',(-0.481096510297973,-0.277761199726725,
0.473510370999757));
#31175=CARTESIAN_POINT('Ctrl Pts',(-0.481444207517858,-0.187589153728889,
0.499366949904929));
#31176=CARTESIAN_POINT('Ctrl Pts',(-0.482123504397716,-0.00973590381621485,
0.528529637179682));
#31177=CARTESIAN_POINT('Ctrl Pts',(-0.481560106591152,0.157531805062946,
0.507985809539986));
#31178=CARTESIAN_POINT('Ctrl Pts',(-0.481096510297974,0.277761199726725,
0.473510370999757));
#31179=CARTESIAN_POINT('',(-0.48168265812218,-0.105573547381759,0.509528465790875));
#31180=CARTESIAN_POINT('',(-0.481671866090386,0.105573308103865,0.509780497494418));
#31181=CARTESIAN_POINT('Ctrl Pts',(-0.481682776226655,-0.105554844793129,
0.509530050599285));
#31182=CARTESIAN_POINT('Ctrl Pts',(-0.482471555403153,-0.0889600413291659,
0.510257198470763));
#31183=CARTESIAN_POINT('Ctrl Pts',(-0.483081002674462,-0.0724019202065436,
0.510808016142969));
#31184=CARTESIAN_POINT('Ctrl Pts',(-0.48350406187927,-0.0558356242392143,
0.511204872441748));
#31185=CARTESIAN_POINT('Ctrl Pts',(-0.483571425521599,-0.0531977758634472,
0.511268063799986));
#31186=CARTESIAN_POINT('Ctrl Pts',(-0.483634059821167,-0.0505596245392988,
0.511327399849453));
#31187=CARTESIAN_POINT('Ctrl Pts',(-0.483691931501727,-0.047920886921818,
0.511383022134839));
#31188=CARTESIAN_POINT('Ctrl Pts',(-0.48377226082532,-0.0442581626687918,
0.511460229164573));
#31189=CARTESIAN_POINT('Ctrl Pts',(-0.483843374961778,-0.0405965669336863,
0.511530213514606));
#31190=CARTESIAN_POINT('Ctrl Pts',(-0.483905237009646,-0.0369355032943481,
0.511593366062782));
#31191=CARTESIAN_POINT('Ctrl Pts',(-0.484023740592018,-0.0299223317052114,
0.511714341740967));
#31192=CARTESIAN_POINT('Ctrl Pts',(-0.484108299964325,-0.0229111484510916,
0.511810232838511));
#31193=CARTESIAN_POINT('Ctrl Pts',(-0.484158788944568,-0.0158973041957685,
0.511878119719765));
#31194=CARTESIAN_POINT('Ctrl Pts',(-0.484221390237341,-0.00720083784635109,
0.511962292672129));
#31195=CARTESIAN_POINT('Ctrl Pts',(-0.484231570102655,0.00149145331024759,
0.512003262320269));
#31196=CARTESIAN_POINT('Ctrl Pts',(-0.484189431542939,0.010188440724828,
0.511996173735513));
#31197=CARTESIAN_POINT('Ctrl Pts',(-0.484141330609844,0.0201160038064456,
0.51198808215518));
#31198=CARTESIAN_POINT('Ctrl Pts',(-0.484025105493291,0.0300394371693865,
0.511917315710112));
#31199=CARTESIAN_POINT('Ctrl Pts',(-0.483841363935383,0.0399715823347925,
0.511778573331064));
#31200=CARTESIAN_POINT('Ctrl Pts',(-0.483530538123121,0.0567732635858149,
0.511543870234205));
#31201=CARTESIAN_POINT('Ctrl Pts',(-0.483027218617348,0.0735601148901351,
0.511114228132524));
#31202=CARTESIAN_POINT('Ctrl Pts',(-0.482337584156177,0.0903849359947383,
0.510480081135851));
#31203=CARTESIAN_POINT('Ctrl Pts',(-0.482131355509923,0.0954162392071141,
0.510290445489704));
#31204=CARTESIAN_POINT('Ctrl Pts',(-0.481908583230074,0.100448074937233,
0.510082742562517));
#31205=CARTESIAN_POINT('Ctrl Pts',(-0.481669499211642,0.105481542418297,
0.509857066299145));
#31206=CARTESIAN_POINT('Ctrl Pts',(-0.481669499211638,0.105481542420091,
0.509857066298925));
#31207=CARTESIAN_POINT('Ctrl Pts',(-0.481542291138614,0.158851785396327,
0.503329833692243));
#31208=CARTESIAN_POINT('Ctrl Pts',(-0.481338736582444,0.214942061649024,
0.491523580997232));
#31209=CARTESIAN_POINT('Ctrl Pts',(-0.481096510297974,0.277761199726725,
0.473510370999757));
#31210=CARTESIAN_POINT('Ctrl Pts',(-0.5,0.267674912507137,0.445024157409747));
#31211=CARTESIAN_POINT('Ctrl Pts',(-0.5,0.150652619934056,0.47744405363793));
#31212=CARTESIAN_POINT('Ctrl Pts',(-0.5,-0.00916398135951556,0.495845869769615));
#31213=CARTESIAN_POINT('Ctrl Pts',(-0.5,-0.180075676750139,0.469283396273211));
#31214=CARTESIAN_POINT('Ctrl Pts',(-0.5,-0.267674925037408,0.44502404899404));
#31215=CARTESIAN_POINT('Ctrl Pts',(-0.481096510297973,-0.277761199726725,
0.473510370999757));
#31216=CARTESIAN_POINT('Ctrl Pts',(-0.481338736582444,-0.214942061649024,
0.491523580997232));
#31217=CARTESIAN_POINT('Ctrl Pts',(-0.481553507568566,-0.158892946912006,
0.503053570640112));
#31218=CARTESIAN_POINT('Ctrl Pts',(-0.481682776226651,-0.105554844794932,
0.509530050599066));
#31219=CARTESIAN_POINT('Ctrl Pts',(0.0164555589739993,0.567849647786322,
0.444468924013264));
#31220=CARTESIAN_POINT('Ctrl Pts',(0.093087014197801,0.523606456484467,
0.469110141953085));
#31221=CARTESIAN_POINT('Ctrl Pts',(0.242091658608015,0.437578584923725,
0.495972649874704));
#31222=CARTESIAN_POINT('Ctrl Pts',(0.381369167394267,0.357166677733922,
0.477323881266358));
#31223=CARTESIAN_POINT('Ctrl Pts',(0.483544441026001,0.298175755998117,
0.444468924013264));
#31224=CARTESIAN_POINT('Ctrl Pts',(0.0109703726493329,0.563740565008697,
0.454149406342095));
#31225=CARTESIAN_POINT('Ctrl Pts',(0.0881463865169628,0.51931680134957,
0.479195744603699));
#31226=CARTESIAN_POINT('Ctrl Pts',(0.238936621724158,0.432519619069652,
0.506818674741199));
#31227=CARTESIAN_POINT('Ctrl Pts',(0.37998164439088,0.350870246231151,0.487544524024234));
#31228=CARTESIAN_POINT('Ctrl Pts',(0.482728464116658,0.291370903907653,
0.454149406342095));
#31229=CARTESIAN_POINT('Ctrl Pts',(0.00548518632466648,0.559631482231073,
0.463829888670926));
#31230=CARTESIAN_POINT('Ctrl Pts',(0.0832057588361247,0.515027146214673,
0.489281347254314));
#31231=CARTESIAN_POINT('Ctrl Pts',(0.235781584840302,0.427460653215579,
0.517664699607693));
#31232=CARTESIAN_POINT('Ctrl Pts',(0.378594121387492,0.344573814728379,
0.49776516678211));
#31233=CARTESIAN_POINT('Ctrl Pts',(0.481912487207316,0.284566051817189,
0.463829888670926));
#31234=CARTESIAN_POINT('Ctrl Pts',(6.93889390390723E-17,0.555522399453449,
0.473510370999757));
#31235=CARTESIAN_POINT('Ctrl Pts',(0.0782651311552866,0.510737491079776,
0.499366949904929));
#31236=CARTESIAN_POINT('Ctrl Pts',(0.232626547956445,0.422401687361506,
0.528510724474188));
#31237=CARTESIAN_POINT('Ctrl Pts',(0.377206598384105,0.338277383225607,
0.507985809539986));
#31238=CARTESIAN_POINT('Ctrl Pts',(0.481096510297974,0.277761199726724,
0.473510370999756));
#31239=CARTESIAN_POINT('',(0.149409184436338,0.469937918404108,0.509521990816289));
#31240=CARTESIAN_POINT('',(0.332265600557506,0.364353270357514,0.509774885821379));
#31241=CARTESIAN_POINT('Ctrl Pts',(0.149426910636359,0.469927842071009,
0.509523338656205));
#31242=CARTESIAN_POINT('Ctrl Pts',(0.16419169647835,0.462314146222986,0.510249567790538));
#31243=CARTESIAN_POINT('Ctrl Pts',(0.178835082930703,0.454563489646878,
0.510799578547905));
#31244=CARTESIAN_POINT('Ctrl Pts',(0.193392414706915,0.446647318723277,
0.511195921402444));
#31245=CARTESIAN_POINT('Ctrl Pts',(0.195711475839183,0.44538623018126,0.511259060947736));
#31246=CARTESIAN_POINT('Ctrl Pts',(0.198028434168209,0.444120890154363,
0.511318349002625));
#31247=CARTESIAN_POINT('Ctrl Pts',(0.200343518860398,0.442851127855779,
0.511373928077867));
#31248=CARTESIAN_POINT('Ctrl Pts',(0.20355567906179,0.441089343531216,0.511451043569201));
#31249=CARTESIAN_POINT('Ctrl Pts',(0.206762257171419,0.439320141024336,
0.511520951504384));
#31250=CARTESIAN_POINT('Ctrl Pts',(0.209963751633228,0.43754318992796,0.511584044834106));
#31251=CARTESIAN_POINT('Ctrl Pts',(0.216096567725542,0.43413924392427,0.511704907072804));
#31252=CARTESIAN_POINT('Ctrl Pts',(0.222210701535505,0.430706887856039,
0.511800747922412));
#31253=CARTESIAN_POINT('Ctrl Pts',(0.228310114954446,0.427243688838005,
0.511868640474087));
#31254=CARTESIAN_POINT('Ctrl Pts',(0.235872778398072,0.422949667952265,
0.511952820457207));
#31255=CARTESIAN_POINT('Ctrl Pts',(0.243405631153963,0.418612326195932,
0.511993883112242));
#31256=CARTESIAN_POINT('Ctrl Pts',(0.250916404544279,0.414227319096577,
0.511986957182662));
#31257=CARTESIAN_POINT('Ctrl Pts',(0.259489910871209,0.409221857720465,
0.511979051272313));
#31258=CARTESIAN_POINT('Ctrl Pts',(0.26802579525337,0.404159453368485,0.511908560978455));
#31259=CARTESIAN_POINT('Ctrl Pts',(0.276535477804989,0.399034214614234,
0.511770158465883));
#31260=CARTESIAN_POINT('Ctrl Pts',(0.290930854775299,0.390364121049316,
0.511536030303048));
#31261=CARTESIAN_POINT('Ctrl Pts',(0.305217174954266,0.381534716705735,
0.511107142930622));
#31262=CARTESIAN_POINT('Ctrl Pts',(0.319443230723362,0.372524966389875,
0.510473800924481));
#31263=CARTESIAN_POINT('Ctrl Pts',(0.323697397804576,0.369830685991582,
0.510284406003119));
#31264=CARTESIAN_POINT('Ctrl Pts',(0.327943755152913,0.367121811453886,
0.510076948258661));
#31265=CARTESIAN_POINT('Ctrl Pts',(0.332183370119856,0.364397994326456,
0.509851518489548));
#31266=CARTESIAN_POINT('Ctrl Pts',(0.332183370121399,0.36439799432556,0.50985151848933));
#31267=CARTESIAN_POINT('Ctrl Pts',(0.3783402555425,0.337602359554229,0.503326883310332));
#31268=CARTESIAN_POINT('Ctrl Pts',(0.426814654021077,0.30938054288139,0.491523580997232));
#31269=CARTESIAN_POINT('Ctrl Pts',(0.481096510297974,0.277761199726724,
0.473510370999756));
#31270=CARTESIAN_POINT('Ctrl Pts',(0.481813273998462,0.299175245747479,
0.44502415632149));
#31271=CARTESIAN_POINT('Ctrl Pts',(0.380468973768911,0.357686404765844,
0.47744392523402));
#31272=CARTESIAN_POINT('Ctrl Pts',(0.242060328974596,0.437596673096014,
0.495826064932766));
#31273=CARTESIAN_POINT('Ctrl Pts',(0.0940498670900422,0.523050553107941,
0.469283267869301));
#31274=CARTESIAN_POINT('Ctrl Pts',(0.0181867147103404,0.566850164555936,
0.445024047543947));
#31275=CARTESIAN_POINT('Ctrl Pts',(6.93889390390723E-17,0.555522399453449,
0.473510370999757));
#31276=CARTESIAN_POINT('Ctrl Pts',(0.0545240825613667,0.524322604530414,
0.491523580997232));
#31277=CARTESIAN_POINT('Ctrl Pts',(0.103170663120928,0.496484571131604,
0.503049636797564));
#31278=CARTESIAN_POINT('Ctrl Pts',(0.149426910634818,0.469927842071894,
0.50952333865599));
#31279=CARTESIAN_POINT('Origin',(-1.56125112837913E-17,0.566850269189626,
0.));
#31280=CARTESIAN_POINT('',(0.0181865334794732,0.566850269189626,0.0531981726275096));
#31281=CARTESIAN_POINT('',(-0.0181865334794732,0.566850269189626,0.0531981726275097));
#31282=CARTESIAN_POINT('Ctrl Pts',(0.0181865334794732,0.566850269189626,
0.0531981726275096));
#31283=CARTESIAN_POINT('Ctrl Pts',(-8.32667268468867E-17,0.566850269189626,
0.0528614692578828));
#31284=CARTESIAN_POINT('Ctrl Pts',(-0.0181865334794732,0.566850269189626,
0.0531981726275097));
#31285=CARTESIAN_POINT('',(-0.0181865334794732,0.566850269189626,0.));
#31286=CARTESIAN_POINT('',(0.0181865334794732,0.566850269189626,0.));
#31287=CARTESIAN_POINT('Origin',(-0.490906733260263,-0.283425134594813,
0.));
#31288=CARTESIAN_POINT('',(-0.5,-0.267675134594813,0.0531981726275096));
#31289=CARTESIAN_POINT('',(-0.481813466520527,-0.299175134594813,0.0531981726275097));
#31290=CARTESIAN_POINT('Ctrl Pts',(-0.5,-0.267675134594813,0.0531981726275096));
#31291=CARTESIAN_POINT('Ctrl Pts',(-0.490906733260263,-0.283425134594813,
0.0528614692578827));
#31292=CARTESIAN_POINT('Ctrl Pts',(-0.481813466520527,-0.299175134594813,
0.0531981726275097));
#31293=CARTESIAN_POINT('',(-0.481813466520527,-0.299175134594813,0.));
#31294=CARTESIAN_POINT('',(-0.5,-0.267675134594813,0.));
#31295=CARTESIAN_POINT('Ctrl Pts',(-0.0164555589739992,-0.567849647786322,
0.444468924013264));
#31296=CARTESIAN_POINT('Ctrl Pts',(-0.118630832605735,-0.508858726050516,
0.477323881266358));
#31297=CARTESIAN_POINT('Ctrl Pts',(-0.257908341391988,-0.428446818860712,
0.495972649874704));
#31298=CARTESIAN_POINT('Ctrl Pts',(-0.4069129858022,-0.342418947299971,
0.469110141953084));
#31299=CARTESIAN_POINT('Ctrl Pts',(-0.483544441026001,-0.298175755998117,
0.444468924013264));
#31300=CARTESIAN_POINT('Ctrl Pts',(-0.0109703726493328,-0.563740565008698,
0.454149406342095));
#31301=CARTESIAN_POINT('Ctrl Pts',(-0.113871724472839,-0.504508880129861,
0.487544524024234));
#31302=CARTESIAN_POINT('Ctrl Pts',(-0.255104666887411,-0.423184993842378,
0.506818674741198));
#31303=CARTESIAN_POINT('Ctrl Pts',(-0.405668349322324,-0.335995410650276,
0.479195744603699));
#31304=CARTESIAN_POINT('Ctrl Pts',(-0.482728464116658,-0.291370903907653,
0.454149406342095));
#31305=CARTESIAN_POINT('Ctrl Pts',(-0.00548518632466635,-0.559631482231073,
0.463829888670926));
#31306=CARTESIAN_POINT('Ctrl Pts',(-0.109112616339944,-0.500159034209207,
0.49776516678211));
#31307=CARTESIAN_POINT('Ctrl Pts',(-0.252300992382833,-0.417923168824045,
0.517664699607693));
#31308=CARTESIAN_POINT('Ctrl Pts',(-0.404423712842448,-0.329571874000581,
0.489281347254314));
#31309=CARTESIAN_POINT('Ctrl Pts',(-0.481912487207316,-0.284566051817189,
0.463829888670926));
#31310=CARTESIAN_POINT('Ctrl Pts',(5.55111512312578E-17,-0.555522399453449,
0.473510370999757));
#31311=CARTESIAN_POINT('Ctrl Pts',(-0.104353508207049,-0.495809188288552,
0.507985809539987));
#31312=CARTESIAN_POINT('Ctrl Pts',(-0.249497317878256,-0.412661343805712,
0.528510724474188));
#31313=CARTESIAN_POINT('Ctrl Pts',(-0.403179076362572,-0.323148337350886,
0.499366949904929));
#31314=CARTESIAN_POINT('Ctrl Pts',(-0.481096510297974,-0.277761199726725,
0.473510370999757));
#31315=CARTESIAN_POINT('',(-0.149406387802817,-0.469927086065238,0.509774885821372));
#31316=CARTESIAN_POINT('',(-0.332273583321351,-0.36436110848265,0.509521990816249));
#31317=CARTESIAN_POINT('Ctrl Pts',(-0.149486235114913,-0.469878234401734,
0.509851518489553));
#31318=CARTESIAN_POINT('Ctrl Pts',(-0.164305299506581,-0.462235914123333,
0.510597417196866));
#31319=CARTESIAN_POINT('Ctrl Pts',(-0.179001946260328,-0.454456869632082,
0.511144655182254));
#31320=CARTESIAN_POINT('Ctrl Pts',(-0.193610659347279,-0.446513425625821,
0.511496368941397));
#31321=CARTESIAN_POINT('Ctrl Pts',(-0.195885616680319,-0.445276424386624,
0.511551139939412));
#31322=CARTESIAN_POINT('Ctrl Pts',(-0.198158519935459,-0.444035387571388,
0.511601214129389));
#31323=CARTESIAN_POINT('Ctrl Pts',(-0.200429580583077,-0.442790159279922,
0.511646650667282));
#31324=CARTESIAN_POINT('Ctrl Pts',(-0.209799043912681,-0.437652858862111,
0.511834103158284));
#31325=CARTESIAN_POINT('Ctrl Pts',(-0.219120102170151,-0.432453709590706,
0.511941841246582));
#31326=CARTESIAN_POINT('Ctrl Pts',(-0.228405904398673,-0.427184085359904,
0.511975832565739));
#31327=CARTESIAN_POINT('Ctrl Pts',(-0.235970467119967,-0.422891251845842,
0.512003523169029));
#31328=CARTESIAN_POINT('Ctrl Pts',(-0.243504550902669,-0.418555670166371,
0.511982313941876));
#31329=CARTESIAN_POINT('Ctrl Pts',(-0.251015753293323,-0.414172765833714,
0.511916847499714));
#31330=CARTESIAN_POINT('Ctrl Pts',(-0.258685985372186,-0.409697065185204,
0.511849994980152));
#31331=CARTESIAN_POINT('Ctrl Pts',(-0.26632524258338,-0.40517616383449,
0.511737089964109));
#31332=CARTESIAN_POINT('Ctrl Pts',(-0.2739416447187,-0.400605543537466,
0.511584033754542));
#31333=CARTESIAN_POINT('Ctrl Pts',(-0.274839066022866,-0.400066998965511,
0.511565999530408));
#31334=CARTESIAN_POINT('Ctrl Pts',(-0.275736168344317,-0.399527764729909,
0.511547408980238));
#31335=CARTESIAN_POINT('Ctrl Pts',(-0.276632964213637,-0.3989878343978,
0.511528252667955));
#31336=CARTESIAN_POINT('Ctrl Pts',(-0.291025308731488,-0.390322692617817,
0.511220820112226));
#31337=CARTESIAN_POINT('Ctrl Pts',(-0.305305244489192,-0.381498545649502,
0.510766837024551));
#31338=CARTESIAN_POINT('Ctrl Pts',(-0.319523357654944,-0.372493888356987,
0.510136230701218));
#31339=CARTESIAN_POINT('Ctrl Pts',(-0.32377514957593,-0.36980113097904,
0.50994765385986));
#31340=CARTESIAN_POINT('Ctrl Pts',(-0.328018991519792,-0.367093762821116,
0.509743503525081));
#31341=CARTESIAN_POINT('Ctrl Pts',(-0.332255993860885,-0.364371421655637,
0.50952333865621));
#31342=CARTESIAN_POINT('Ctrl Pts',(-0.332255993862454,-0.364371421654726,
0.50952333865599));
#31343=CARTESIAN_POINT('Ctrl Pts',(-0.378382919626528,-0.337590700753811,
0.503049636797564));
#31344=CARTESIAN_POINT('Ctrl Pts',(-0.426814654021078,-0.30938054288139,
0.491523580997232));
#31345=CARTESIAN_POINT('Ctrl Pts',(-0.481096510297974,-0.277761199726725,
0.473510370999757));
#31346=CARTESIAN_POINT('Ctrl Pts',(-0.481813285289703,-0.299175239228478,
0.445024047543933));
#31347=CARTESIAN_POINT('Ctrl Pts',(-0.405950132909983,-0.342974850676483,
0.469283267869296));
#31348=CARTESIAN_POINT('Ctrl Pts',(-0.257939671025431,-0.42842873068841,
0.495826064932765));
#31349=CARTESIAN_POINT('Ctrl Pts',(-0.119531026231113,-0.508338999018581,
0.477443925234023));
#31350=CARTESIAN_POINT('Ctrl Pts',(-0.0181867260015819,-0.566850158036935,
0.445024156321504));
#31351=CARTESIAN_POINT('Ctrl Pts',(5.55111512312578E-17,-0.555522399453449,
0.473510370999757));
#31352=CARTESIAN_POINT('Ctrl Pts',(-0.0545240825613664,-0.524322604530414,
0.491523580997232));
#31353=CARTESIAN_POINT('Ctrl Pts',(-0.103202091980281,-0.496453452351216,
0.503326883310332));
#31354=CARTESIAN_POINT('Ctrl Pts',(-0.149486235113333,-0.46987823440264,
0.50985151848933));
#31355=CARTESIAN_POINT('Ctrl Pts',(0.5,0.269673891788205,0.444468924013264));
#31356=CARTESIAN_POINT('Ctrl Pts',(0.5,0.151692048316592,0.477323881266358));
#31357=CARTESIAN_POINT('Ctrl Pts',(0.5,-0.00912777933363709,0.495992583115463));
#31358=CARTESIAN_POINT('Ctrl Pts',(0.5,-0.181187509184497,0.469110141953084));
#31359=CARTESIAN_POINT('Ctrl Pts',(0.5,-0.269673891788205,0.444468924013264));
#31360=CARTESIAN_POINT('Ctrl Pts',(0.493698836765991,0.272369661101045,
0.454149406342095));
#31361=CARTESIAN_POINT('Ctrl Pts',(0.493853368863718,0.153638633898709,
0.487544524024234));
#31362=CARTESIAN_POINT('Ctrl Pts',(0.494041168132572,-0.00933048749449758,
0.506838267803537));
#31363=CARTESIAN_POINT('Ctrl Pts',(0.493814735839286,-0.183321390699295,
0.479195744603699));
#31364=CARTESIAN_POINT('Ctrl Pts',(0.493698836765991,-0.272369661101045,
0.454149406342095));
#31365=CARTESIAN_POINT('Ctrl Pts',(0.487397673531982,0.275065430413885,
0.463829888670926));
#31366=CARTESIAN_POINT('Ctrl Pts',(0.487706737727435,0.155585219480827,
0.49776516678211));
#31367=CARTESIAN_POINT('Ctrl Pts',(0.488082336265144,-0.00953319565535789,
0.517683952491609));
#31368=CARTESIAN_POINT('Ctrl Pts',(0.487629471678572,-0.185455272214093,
0.489281347254314));
#31369=CARTESIAN_POINT('Ctrl Pts',(0.487397673531982,-0.275065430413885,
0.463829888670926));
#31370=CARTESIAN_POINT('Ctrl Pts',(0.481096510297974,0.277761199726725,
0.473510370999757));
#31371=CARTESIAN_POINT('Ctrl Pts',(0.481560106591153,0.157531805062944,
0.507985809539987));
#31372=CARTESIAN_POINT('Ctrl Pts',(0.482123504397716,-0.00973590381621833,
0.528529637179682));
#31373=CARTESIAN_POINT('Ctrl Pts',(0.481444207517858,-0.187589153728891,
0.499366949904929));
#31374=CARTESIAN_POINT('Ctrl Pts',(0.481096510297973,-0.277761199726725,
0.473510370999756));
#31375=CARTESIAN_POINT('',(0.481671866090396,0.105573308103687,0.509780497494203));
#31376=CARTESIAN_POINT('',(0.484214864131698,-5.47020833232433E-5,0.511982600478171));
#31377=CARTESIAN_POINT('Ctrl Pts',(0.481669499211642,0.105481542418299,
0.509857066299145));
#31378=CARTESIAN_POINT('Ctrl Pts',(0.482460593225416,0.0888265354508503,
0.510603796014394));
#31379=CARTESIAN_POINT('Ctrl Pts',(0.483072065647681,0.0722091798017497,
0.511151842975794));
#31380=CARTESIAN_POINT('Ctrl Pts',(0.483497190939341,0.0555857456715263,
0.511504223118381));
#31381=CARTESIAN_POINT('Ctrl Pts',(0.483563383885825,0.0529974402769593,
0.511559089484552));
#31382=CARTESIAN_POINT('Ctrl Pts',(0.483625056117804,0.0504088952732917,
0.511609256996307));
#31383=CARTESIAN_POINT('Ctrl Pts',(0.4836821783703,0.047819849573354,0.511654784300019));
#31384=CARTESIAN_POINT('Ctrl Pts',(0.483917872556838,0.0371370947188088,
0.511842636150125));
#31385=CARTESIAN_POINT('Ctrl Pts',(0.484075802257484,0.0264653210899992,
0.511950708373913));
#31386=CARTESIAN_POINT('Ctrl Pts',(0.484155071769149,0.0157888211313803,
0.511984934956568));
#31387=CARTESIAN_POINT('Ctrl Pts',(0.484194291677581,0.0105064453231446,
0.512001869127216));
#31388=CARTESIAN_POINT('Ctrl Pts',(0.48421423214258,0.00522594818450658,
0.512000762646226));
#31389=CARTESIAN_POINT('Ctrl Pts',(0.484214864131698,-5.47020833232433E-5,
0.511982600478171));
#31390=CARTESIAN_POINT('',(0.481681895506807,-0.105694312340346,0.509518232484153));
#31391=CARTESIAN_POINT('Ctrl Pts',(0.484214864131698,-5.47020833232433E-5,
0.511982600478171));
#31392=CARTESIAN_POINT('Ctrl Pts',(0.484215270731505,-0.00346871674032279,
0.511970861826781));
#31393=CARTESIAN_POINT('Ctrl Pts',(0.484207605431539,-0.00688277797801751,
0.511951999455987));
#31394=CARTESIAN_POINT('Ctrl Pts',(0.484191857341194,-0.0102974597917216,
0.511926310507199));
#31395=CARTESIAN_POINT('Ctrl Pts',(0.484150901779444,-0.0191779150605256,
0.511859502068503));
#31396=CARTESIAN_POINT('Ctrl Pts',(0.484055314691237,-0.0280541644854541,
0.511746554850449));
#31397=CARTESIAN_POINT('Ctrl Pts',(0.483905243422272,-0.0369355028308617,
0.511593354983391));
#31398=CARTESIAN_POINT('Ctrl Pts',(0.483887560906102,-0.0379819683534304,
0.511575303832461));
#31399=CARTESIAN_POINT('Ctrl Pts',(0.483869121649569,-0.0390285027730886,
0.511556694950178));
#31400=CARTESIAN_POINT('Ctrl Pts',(0.483849926346507,-0.0400751201476585,
0.51153751894854));
#31401=CARTESIAN_POINT('Ctrl Pts',(0.483541868042211,-0.0568718944734031,
0.511229770405657));
#31402=CARTESIAN_POINT('Ctrl Pts',(0.483039907069928,-0.0736508998392528,
0.510775123483089));
#31403=CARTESIAN_POINT('Ctrl Pts',(0.482350711259662,-0.0904666554307169,
0.510143705463836));
#31404=CARTESIAN_POINT('Ctrl Pts',(0.482144613787803,-0.0954952476873488,
0.50995488589251));
#31405=CARTESIAN_POINT('Ctrl Pts',(0.481921888290475,-0.100524263582078,
0.509750479628641));
#31406=CARTESIAN_POINT('Ctrl Pts',(0.481682776226655,-0.10555484479313,
0.509530050599285));
#31407=CARTESIAN_POINT('Ctrl Pts',(0.481682776226651,-0.105554844794933,
0.509530050599066));
#31408=CARTESIAN_POINT('Ctrl Pts',(0.481553507568566,-0.158892946912007,
0.503053570640112));
#31409=CARTESIAN_POINT('Ctrl Pts',(0.481338736582444,-0.214942061649024,
0.491523580997232));
#31410=CARTESIAN_POINT('Ctrl Pts',(0.481096510297973,-0.277761199726725,
0.473510370999756));
#31411=CARTESIAN_POINT('Ctrl Pts',(0.5,-0.267674925037459,0.445024048994026));
#31412=CARTESIAN_POINT('Ctrl Pts',(0.5,-0.180075676750169,0.469283396273207));
#31413=CARTESIAN_POINT('Ctrl Pts',(0.5,-0.00916398135954615,0.495845869769614));
#31414=CARTESIAN_POINT('Ctrl Pts',(0.5,0.150652619934028,0.477444053637933));
#31415=CARTESIAN_POINT('Ctrl Pts',(0.5,0.267674912507086,0.445024157409761));
#31416=CARTESIAN_POINT('Ctrl Pts',(0.481096510297974,0.277761199726725,
0.473510370999757));
#31417=CARTESIAN_POINT('Ctrl Pts',(0.481338736582444,0.214942061649024,
0.491523580997232));
#31418=CARTESIAN_POINT('Ctrl Pts',(0.481542291138614,0.158851785396327,
0.503329833692243));
#31419=CARTESIAN_POINT('Ctrl Pts',(0.481669499211638,0.105481542420091,
0.509857066298925));
#31420=CARTESIAN_POINT('Origin',(0.490906733260264,0.283425134594813,0.));
#31421=CARTESIAN_POINT('',(0.5,0.267675134594813,0.0531981726275096));
#31422=CARTESIAN_POINT('',(0.481813466520527,0.299175134594813,0.0531981726275097));
#31423=CARTESIAN_POINT('Ctrl Pts',(0.5,0.267675134594813,0.0531981726275096));
#31424=CARTESIAN_POINT('Ctrl Pts',(0.490906733260264,0.283425134594813,
0.0528614692578827));
#31425=CARTESIAN_POINT('Ctrl Pts',(0.481813466520527,0.299175134594813,
0.0531981726275097));
#31426=CARTESIAN_POINT('',(0.481813466520527,0.299175134594813,0.));
#31427=CARTESIAN_POINT('',(0.5,0.267675134594813,0.));
#31428=CARTESIAN_POINT('Origin',(-1.37043154602168E-16,-0.566850269189626,
0.));
#31429=CARTESIAN_POINT('',(-0.0181865334794733,-0.566850269189626,0.0531981726275096));
#31430=CARTESIAN_POINT('',(0.018186533479473,-0.566850269189626,0.0531981726275097));
#31431=CARTESIAN_POINT('Ctrl Pts',(-0.0181865334794733,-0.566850269189626,
0.0531981726275096));
#31432=CARTESIAN_POINT('Ctrl Pts',(-9.71445146547012E-17,-0.566850269189626,
0.0528614692578828));
#31433=CARTESIAN_POINT('Ctrl Pts',(0.018186533479473,-0.566850269189626,
0.0531981726275097));
#31434=CARTESIAN_POINT('',(0.018186533479473,-0.566850269189626,0.));
#31435=CARTESIAN_POINT('',(-0.0181865334794733,-0.566850269189626,0.));
#31436=CARTESIAN_POINT('Ctrl Pts',(0.483544441026,-0.298175755998118,0.444468924013264));
#31437=CARTESIAN_POINT('Ctrl Pts',(0.406912985802199,-0.342418947299972,
0.469110141953084));
#31438=CARTESIAN_POINT('Ctrl Pts',(0.257908341391985,-0.428446818860714,
0.495972649874704));
#31439=CARTESIAN_POINT('Ctrl Pts',(0.118630832605733,-0.508858726050517,
0.477323881266358));
#31440=CARTESIAN_POINT('Ctrl Pts',(0.0164555589739991,-0.567849647786322,
0.444468924013264));
#31441=CARTESIAN_POINT('Ctrl Pts',(0.482728464116658,-0.291370903907653,
0.454149406342095));
#31442=CARTESIAN_POINT('Ctrl Pts',(0.405668349322323,-0.335995410650277,
0.479195744603699));
#31443=CARTESIAN_POINT('Ctrl Pts',(0.255104666887408,-0.42318499384238,
0.506818674741198));
#31444=CARTESIAN_POINT('Ctrl Pts',(0.113871724472837,-0.504508880129862,
0.487544524024234));
#31445=CARTESIAN_POINT('Ctrl Pts',(0.0109703726493327,-0.563740565008698,
0.454149406342095));
#31446=CARTESIAN_POINT('Ctrl Pts',(0.481912487207315,-0.284566051817189,
0.463829888670926));
#31447=CARTESIAN_POINT('Ctrl Pts',(0.404423712842447,-0.329571874000583,
0.489281347254314));
#31448=CARTESIAN_POINT('Ctrl Pts',(0.252300992382831,-0.417923168824047,
0.517664699607693));
#31449=CARTESIAN_POINT('Ctrl Pts',(0.109112616339942,-0.500159034209208,
0.49776516678211));
#31450=CARTESIAN_POINT('Ctrl Pts',(0.00548518632466623,-0.559631482231073,
0.463829888670926));
#31451=CARTESIAN_POINT('Ctrl Pts',(0.481096510297973,-0.277761199726725,
0.473510370999757));
#31452=CARTESIAN_POINT('Ctrl Pts',(0.403179076362571,-0.323148337350888,
0.499366949904929));
#31453=CARTESIAN_POINT('Ctrl Pts',(0.249497317878254,-0.412661343805714,
0.528510724474188));
#31454=CARTESIAN_POINT('Ctrl Pts',(0.104353508207047,-0.495809188288553,
0.507985809539986));
#31455=CARTESIAN_POINT('Ctrl Pts',(-1.94289029309402E-16,-0.555522399453449,
0.473510370999756));
#31456=CARTESIAN_POINT('',(0.332273583321351,-0.364361108482647,0.509521990816293));
#31457=CARTESIAN_POINT('',(0.14940638780266,-0.469927086065317,0.509774885821586));
#31458=CARTESIAN_POINT('Ctrl Pts',(0.332255993860884,-0.364371421655637,
0.50952333865621));
#31459=CARTESIAN_POINT('Ctrl Pts',(0.318279946918772,-0.373351253352252,
0.510249567790544));
#31460=CARTESIAN_POINT('Ctrl Pts',(0.30424598820164,-0.382157469729392,
0.510799578547912));
#31461=CARTESIAN_POINT('Ctrl Pts',(0.290111717192956,-0.390806403397131,
0.511195921402451));
#31462=CARTESIAN_POINT('Ctrl Pts',(0.28786005191306,-0.392184224979568,
0.511259060947741));
#31463=CARTESIAN_POINT('Ctrl Pts',(0.285605756140875,-0.393558099738538,
0.51131834900263));
#31464=CARTESIAN_POINT('Ctrl Pts',(0.283348567387484,-0.394928140744567,
0.51137392807787));
#31465=CARTESIAN_POINT('Ctrl Pts',(0.28021673730573,-0.396829060917713,
0.511451043569204));
#31466=CARTESIAN_POINT('Ctrl Pts',(0.277081273935522,-0.39872143776643,
0.511520951504387));
#31467=CARTESIAN_POINT('Ctrl Pts',(0.273941641913878,-0.400605537752241,
0.511584044834109));
#31468=CARTESIAN_POINT('Ctrl Pts',(0.267927330155411,-0.40421473928308,
0.511704907072807));
#31469=CARTESIAN_POINT('Ctrl Pts',(0.261897755700506,-0.407793556450531,
0.511800747922414));
#31470=CARTESIAN_POINT('Ctrl Pts',(0.255848830663054,-0.411344203910501,
0.51186864047409));
#31471=CARTESIAN_POINT('Ctrl Pts',(0.248348767769807,-0.415746652130085,
0.51195282045721));
#31472=CARTESIAN_POINT('Ctrl Pts',(0.240826093245984,-0.420101623101487,
0.511993883112245));
#31473=CARTESIAN_POINT('Ctrl Pts',(0.23327317900701,-0.42441364010989,0.511986957182665));
#31474=CARTESIAN_POINT('Ctrl Pts',(0.224651569134172,-0.429335783700461,
0.511979051272316));
#31475=CARTESIAN_POINT('Ctrl Pts',(0.215999456170051,-0.434196874243189,
0.511908560978458));
#31476=CARTESIAN_POINT('Ctrl Pts',(0.207306027932593,-0.43900385613391,
0.511770158465886));
#31477=CARTESIAN_POINT('Ctrl Pts',(0.192599818167027,-0.447135571504794,
0.511536030303051));
#31478=CARTESIAN_POINT('Ctrl Pts',(0.177810169615715,-0.455093185534589,
0.511107142930624));
#31479=CARTESIAN_POINT('Ctrl Pts',(0.162894469075872,-0.462908436068353,
0.510473800924483));
#31480=CARTESIAN_POINT('Ctrl Pts',(0.158434070265442,-0.465245512633472,
0.510284406003122));
#31481=CARTESIAN_POINT('Ctrl Pts',(0.153964937425981,-0.467568528701822,
0.510076948258664));
#31482=CARTESIAN_POINT('Ctrl Pts',(0.149486235114913,-0.469878234401733,
0.509851518489553));
#31483=CARTESIAN_POINT('Ctrl Pts',(0.149486235113333,-0.469878234402641,
0.50985151848933));
#31484=CARTESIAN_POINT('Ctrl Pts',(0.10320209198028,-0.496453452351217,
0.503326883310332));
#31485=CARTESIAN_POINT('Ctrl Pts',(0.054524082561366,-0.524322604530415,
0.491523580997232));
#31486=CARTESIAN_POINT('Ctrl Pts',(-1.94289029309402E-16,-0.555522399453449,
0.473510370999756));
#31487=CARTESIAN_POINT('Ctrl Pts',(0.018186726001538,-0.56685015803696,
0.44502415632149));
#31488=CARTESIAN_POINT('Ctrl Pts',(0.119531026231088,-0.508338999018595,
0.47744392523402));
#31489=CARTESIAN_POINT('Ctrl Pts',(0.257939671025404,-0.428428730688425,
0.495826064932766));
#31490=CARTESIAN_POINT('Ctrl Pts',(0.405950132909958,-0.342974850676498,
0.4692832678693));
#31491=CARTESIAN_POINT('Ctrl Pts',(0.481813285289659,-0.299175239228503,
0.445024047543947));
#31492=CARTESIAN_POINT('Ctrl Pts',(0.481096510297973,-0.277761199726725,
0.473510370999757));
#31493=CARTESIAN_POINT('Ctrl Pts',(0.426814654021077,-0.309380542881391,
0.491523580997232));
#31494=CARTESIAN_POINT('Ctrl Pts',(0.378382919626527,-0.337590700753812,
0.503049636797564));
#31495=CARTESIAN_POINT('Ctrl Pts',(0.332255993862453,-0.364371421654726,
0.50952333865599));
#31496=CARTESIAN_POINT('Origin',(0.490906733260263,-0.283425134594813,0.));
#31497=CARTESIAN_POINT('',(0.481813466520527,-0.299175134594813,0.0531981726275097));
#31498=CARTESIAN_POINT('',(0.5,-0.267675134594813,0.0531981726275096));
#31499=CARTESIAN_POINT('Ctrl Pts',(0.481813466520527,-0.299175134594813,
0.0531981726275097));
#31500=CARTESIAN_POINT('Ctrl Pts',(0.490906733260263,-0.283425134594813,
0.0528614692578827));
#31501=CARTESIAN_POINT('Ctrl Pts',(0.5,-0.267675134594813,0.0531981726275096));
#31502=CARTESIAN_POINT('',(0.5,-0.267675134594813,0.));
#31503=CARTESIAN_POINT('',(0.481813466520527,-0.299175134594813,0.));
#31504=CARTESIAN_POINT('Origin',(0.5,0.288675134594813,0.));
#31505=CARTESIAN_POINT('Ctrl Pts',(0.481813466520527,0.299175134594813,
0.0531981726275097));
#31506=CARTESIAN_POINT('Ctrl Pts',(0.249999999999998,0.433012701892221,
-0.0197414764085334));
#31507=CARTESIAN_POINT('Ctrl Pts',(0.0181865334794731,0.566850269189626,
0.0531981726275097));
#31508=CARTESIAN_POINT('Origin',(0.5,-0.288675134594813,0.));
#31509=CARTESIAN_POINT('Ctrl Pts',(0.5,-0.267675134594813,0.0531981726275096));
#31510=CARTESIAN_POINT('Ctrl Pts',(0.5,1.72084568816899E-15,-0.0197414764085334));
#31511=CARTESIAN_POINT('Ctrl Pts',(0.5,0.267675134594813,0.0531981726275096));
#31512=CARTESIAN_POINT('Origin',(-1.06057523872491E-16,-0.577350269189626,
0.));
#31513=CARTESIAN_POINT('Ctrl Pts',(0.018186533479473,-0.566850269189626,
0.0531981726275097));
#31514=CARTESIAN_POINT('Ctrl Pts',(0.250000000000002,-0.433012701892218,
-0.0197414764085333));
#31515=CARTESIAN_POINT('Ctrl Pts',(0.481813466520527,-0.299175134594813,
0.0531981726275097));
#31516=CARTESIAN_POINT('Origin',(0.,0.,0.0439797344638712));
#31517=CARTESIAN_POINT('',(-0.475,-5.81707229594992E-17,-5.55111512312578E-17));
#31518=CARTESIAN_POINT('Origin',(0.,0.,0.));
#31519=CARTESIAN_POINT('',(-0.5,-9.83216870916981E-17,0.0144337567297442));
#31520=CARTESIAN_POINT('',(-0.551175134594813,-6.74994864351149E-17,0.0439797344638712));
#31521=CARTESIAN_POINT('Ctrl Pts',(-0.5,0.267675134594813,0.0531981726275097));
#31522=CARTESIAN_POINT('Ctrl Pts',(-0.5,0.125416837769224,0.0144337567297444));
#31523=CARTESIAN_POINT('Ctrl Pts',(-0.5,-1.35411034226029E-16,0.0144337567297442));
#31524=CARTESIAN_POINT('Ctrl Pts',(-0.0181865334794732,0.566850269189626,
0.0531981726275097));
#31525=CARTESIAN_POINT('Ctrl Pts',(-0.250000000000002,0.433012701892218,
-0.0197414764085335));
#31526=CARTESIAN_POINT('Ctrl Pts',(-0.481813466520527,0.299175134594813,
0.0531981726275096));
#31527=CARTESIAN_POINT('Ctrl Pts',(-0.481813466520527,-0.299175134594813,
0.0531981726275097));
#31528=CARTESIAN_POINT('Ctrl Pts',(-0.249999999999999,-0.43301270189222,
-0.0197414764085333));
#31529=CARTESIAN_POINT('Ctrl Pts',(-0.0181865334794733,-0.566850269189626,
0.0531981726275096));
#31530=CARTESIAN_POINT('Ctrl Pts',(-0.5,-1.35411034226029E-16,0.0144337567297442));
#31531=CARTESIAN_POINT('Ctrl Pts',(-0.5,-0.125416837769225,0.014433756729744));
#31532=CARTESIAN_POINT('Ctrl Pts',(-0.5,-0.267675134594813,0.0531981726275096));
#31533=CARTESIAN_POINT('Origin',(0.,0.,0.476020265536129));
#31534=CARTESIAN_POINT('Origin',(0.,-3.01989654804108E-17,0.5095));
#31535=CARTESIAN_POINT('Origin',(0.,0.,0.476020265536129));
#31536=CARTESIAN_POINT('Origin',(0.,-3.01989654804108E-17,0.5095));
#31537=CARTESIAN_POINT('Origin',(0.,0.,0.476020265536129));
#31538=CARTESIAN_POINT('Origin',(0.,-3.01989654804108E-17,0.5095));
#31539=CARTESIAN_POINT('Origin',(0.,0.,0.476020265536129));
#31540=CARTESIAN_POINT('Origin',(0.,-3.01989654804108E-17,0.5095));
#31541=CARTESIAN_POINT('Origin',(0.,0.,0.476020265536129));
#31542=CARTESIAN_POINT('Origin',(0.,-3.01989654804108E-17,0.5095));
#31543=CARTESIAN_POINT('Origin',(0.,0.,0.476020265536129));
#31544=CARTESIAN_POINT('Origin',(0.,-3.01989654804108E-17,0.5095));
#31545=CARTESIAN_POINT('Origin',(0.,-1.50994827402054E-17,0.51475));
#31546=CARTESIAN_POINT('',(0.454,-5.55989646812898E-17,0.52));
#31547=CARTESIAN_POINT('Origin',(0.,0.,0.52));
#31548=CARTESIAN_POINT('',(0.473593266739736,5.79984478210557E-17,0.51475));
#31549=CARTESIAN_POINT('Origin',(0.,0.,0.52));
#31550=CARTESIAN_POINT('',(-0.366,-4.48220728487931E-17,0.52));
#31551=CARTESIAN_POINT('Origin',(0.,0.,0.52));
#31552=CARTESIAN_POINT('Origin',(0.,-1.01079517131223E-17,0.512575378797541));
#31553=CARTESIAN_POINT('',(-0.330150757595083,6.16297582203915E-33,0.505150757595083));
#31554=CARTESIAN_POINT('Origin',(0.,-2.02159034262446E-17,0.505150757595083));
#31555=CARTESIAN_POINT('',(-0.348075378797541,2.24110364243966E-17,0.512575378797541));
#31556=CARTESIAN_POINT('Origin',(0.,0.,0.5));
#31557=CARTESIAN_POINT('',(-0.319849242404917,-7.83404701841776E-17,0.494849242404917));
#31558=CARTESIAN_POINT('',(-0.325,-3.9801020972289E-17,0.5));
#31559=CARTESIAN_POINT('Origin',(0.,-1.95851175460444E-17,0.494849242404917));
#31560=CARTESIAN_POINT('Origin',(0.,-9.7925587730222E-18,0.476924621202459));
#31561=CARTESIAN_POINT('',(-0.305,3.73517273739943E-17,0.459));
#31562=CARTESIAN_POINT('',(-0.312424621202459,-5.78460987790859E-17,0.476924621202459));
#31563=CARTESIAN_POINT('Origin',(0.,0.,0.459));
#31564=CARTESIAN_POINT('Origin',(0.,0.,0.));
#31565=CARTESIAN_POINT('',(-0.305,-3.73517273739943E-17,0.04));
#31566=CARTESIAN_POINT('',(-0.305,-3.73517273739943E-17,0.));
#31567=CARTESIAN_POINT('Origin',(0.,0.,0.04));
#31568=CARTESIAN_POINT('Origin',(0.,0.,0.02));
#31569=CARTESIAN_POINT('',(-0.345,4.22503145705837E-17,0.));
#31570=CARTESIAN_POINT('',(-0.325,-3.9801020972289E-17,0.02));
#31571=CARTESIAN_POINT('Origin',(0.,0.,0.));
#31572=CARTESIAN_POINT('Origin',(0.,0.,0.));
#31573=CARTESIAN_POINT('Origin',(-0.5,-0.288675134594813,0.));
#31574=CARTESIAN_POINT('Origin',(-0.5,0.288675134594813,0.));
#31575=CARTESIAN_POINT('Origin',(3.53525079574969E-17,0.577350269189626,
0.));
#31624=UNCERTAINTY_MEASURE_WITH_UNIT(LENGTH_MEASURE(0.001),#31639,
'DISTANCE_ACCURACY_VALUE',
'Maximum model space distance between geometric entities at asserted c
onnectivities');
#31625=UNCERTAINTY_MEASURE_WITH_UNIT(LENGTH_MEASURE(0.001),#31639,
'DISTANCE_ACCURACY_VALUE',
'Maximum model space distance between geometric entities at asserted c
onnectivities');
#31637=(
GEOMETRIC_REPRESENTATION_CONTEXT(3)
GLOBAL_UNCERTAINTY_ASSIGNED_CONTEXT((#31624))
GLOBAL_UNIT_ASSIGNED_CONTEXT((#31639,#31641,#31642))
REPRESENTATION_CONTEXT('','3D')
);
#31638=(
GEOMETRIC_REPRESENTATION_CONTEXT(3)
GLOBAL_UNCERTAINTY_ASSIGNED_CONTEXT((#31625))
GLOBAL_UNIT_ASSIGNED_CONTEXT((#31639,#31641,#31642))
REPRESENTATION_CONTEXT('','3D')
);
#31639=(
LENGTH_UNIT()
NAMED_UNIT(*)
SI_UNIT(.CENTI.,.METRE.)
);
#31641=(
NAMED_UNIT(*)
PLANE_ANGLE_UNIT()
SI_UNIT($,.RADIAN.)
);
#31642=(
NAMED_UNIT(*)
SI_UNIT($,.STERADIAN.)
SOLID_ANGLE_UNIT()
);
#31654=SHAPE_DEFINITION_REPRESENTATION(#31666,#31715);
#31666=PRODUCT_DEFINITION_SHAPE('',$,#31728);
#31715=SHAPE_REPRESENTATION('',(#13535),#31637);
#31716=PRODUCT_DEFINITION_CONTEXT('part definition',#31754,'design');
#31728=PRODUCT_DEFINITION('2026-10-22-02-42-33-605',
'11_ISO_4032_M6-8_Hex_Nut',#31740,#31716);
#31740=PRODUCT_DEFINITION_FORMATION('',$,#31767);
#31754=APPLICATION_CONTEXT(
'Core Data for Automotive Mechanical Design Process');
#31755=PRODUCT_CONTEXT('part definition',#31754,'mechanical');
#31767=PRODUCT('2026-10-22-02-42-33-605','11_ISO_4032_M6-8_Hex_Nut',$,(#31755));
#31831=COLOUR_RGB('Black',0.12,0.14,0.17);
#31832=FILL_AREA_STYLE_COLOUR('',#31831);
#31833=FILL_AREA_STYLE('',(#31832));
#31834=SURFACE_STYLE_FILL_AREA(#31833);
#31835=SURFACE_SIDE_STYLE('',(#31834));
#31836=SURFACE_STYLE_USAGE(.BOTH.,#31835);
#31837=PRESENTATION_STYLE_ASSIGNMENT((#31836));
ENDSEC;
END-ISO-10303-21;
